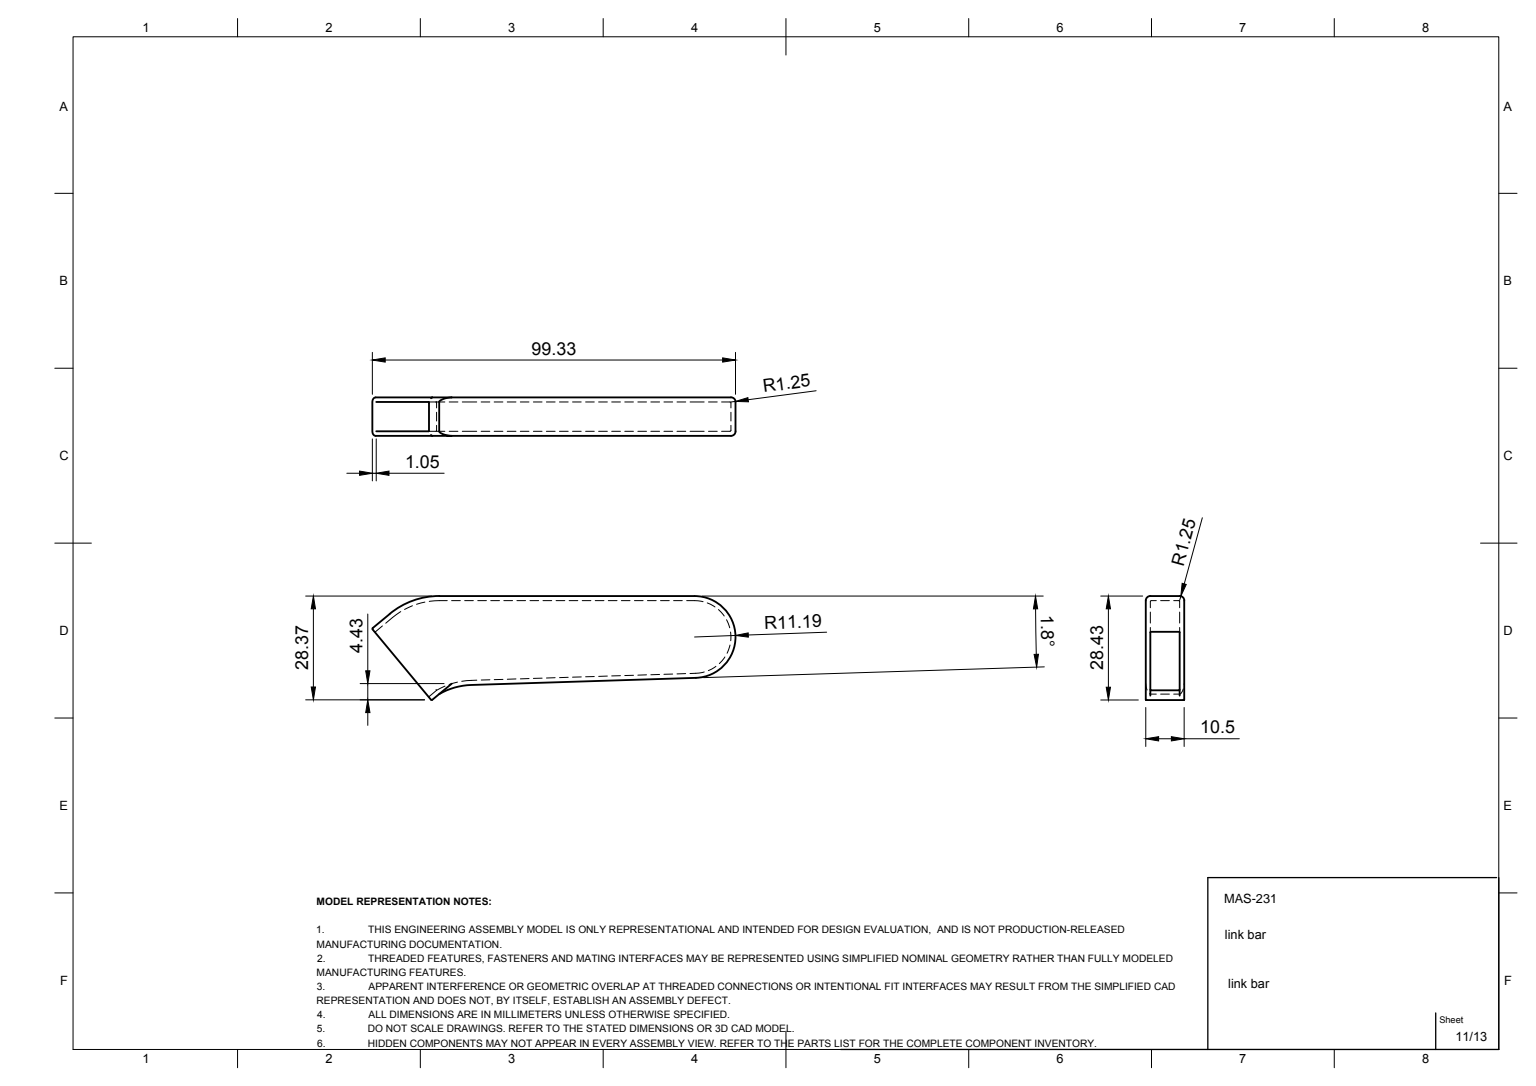
ISO-10303-21;
HEADER;
FILE_DESCRIPTION (('STEP AP214'),
    '1' );
FILE_NAME ( 'Link Bar.step', '2026-10-04T02:08:54', ( '' ), ( '' ), 'STEP AP214', 'Unspecified', '' );
FILE_SCHEMA (( 'AUTOMOTIVE_DESIGN' ));
ENDSEC;
DATA;
#67=ORIENTED_EDGE ( 'NONE', *, *, #18348, .F. ) ;
#85=CARTESIAN_POINT ( 'NONE',  ( 0.1574803149606300023, 0.3648440108500937140, -3.619166627704267558 ) ) ;
#87=CARTESIAN_POINT ( 'NONE',  ( -0.1574803149606299191, 0.7443365962042343131, -3.964450923140766303 ) ) ;
#136=DIRECTION ( 'NONE',  ( -1.000000000000000000, 0.000000000000000000, 0.000000000000000000 ) ) ;
#145=DIRECTION ( 'NONE',  ( 0.000000000000000000, -0.6156614753256641759, -0.7880107536067173513 ) ) ;
#156=DIRECTION ( 'NONE',  ( 0.000000000000000000, 0.6156614753256598460, 0.7880107536067207930 ) ) ;
#159=TOROIDAL_SURFACE ( 'NONE', #46862, 0.3814023619577306956, 0.009842519685039369942 ) ;
#264=EDGE_CURVE ( 'NONE', #24192, #11278, #27216, .T. ) ;
#266=CARTESIAN_POINT ( 'NONE',  ( 0.1673228346456693549, 0.05639690512153990726, -0.1570009270184611616 ) ) ;
#303=EDGE_LOOP ( 'NONE', ( #910, #27362, #9795, #24309 ) ) ;
#308=ORIENTED_EDGE ( 'NONE', *, *, #11008, .T. ) ;
#310=DIRECTION ( 'NONE',  ( 0.000000000000000000, 0.000000000000000000, 1.000000000000000000 ) ) ;
#323=DIRECTION ( 'NONE',  ( -2.602085213965207486E-14, -0.6156614753256566264, -0.7880107536067233465 ) ) ;
#346=CARTESIAN_POINT ( 'NONE',  ( -0.1992661408232795639, -0.3637244504922588773, -1.027838479691305595 ) ) ;
#389=CARTESIAN_POINT ( 'NONE',  ( -0.1673228346456692994, -0.4812165006432425063, -0.8611016091043821596 ) ) ;
#406=DIRECTION ( 'NONE',  ( 0.000000000000000000, -0.2126700594527834443, 0.9771240687918547607 ) ) ;
#428=AXIS2_PLACEMENT_3D ( 'NONE', #42726, #2726, #24548 ) ;
#442=DIRECTION ( 'NONE',  ( 0.000000000000000000, -0.6156614753256597350, -0.7880107536067206819 ) ) ;
#481=ORIENTED_EDGE ( 'NONE', *, *, #44567, .F. ) ;
#483=EDGE_CURVE ( 'NONE', #12524, #45117, #9920, .T. ) ;
#495=FACE_OUTER_BOUND ( 'NONE', #27170, .T. ) ;
#507=CARTESIAN_POINT ( 'NONE',  ( 0.1574803149606300023, -1.308580299410598613, -1.920078980116132872 ) ) ;
#556=DIRECTION ( 'NONE',  ( 0.000000000000000000, 0.9699617890481115889, 0.2432573283306930789 ) ) ;
#568=CARTESIAN_POINT ( 'NONE',  ( -0.2066929133858267931, -0.3022687907404924545, -1.075852903322848331 ) ) ;
#618=DIRECTION ( 'NONE',  ( -0.000000000000000000, 0.7880107536067184615, -0.6156614753256628436 ) ) ;
#643=FACE_OUTER_BOUND ( 'NONE', #21090, .T. ) ;
#670=DIRECTION ( 'NONE',  ( 1.000000000000000000, 0.000000000000000000, -0.000000000000000000 ) ) ;
#700=ORIENTED_EDGE ( 'NONE', *, *, #15382, .F. ) ;
#702=CARTESIAN_POINT ( 'NONE',  ( 0.1925235483212767162, -0.3878655561654137385, -1.008977380820889946 ) ) ;
#751=ORIENTED_EDGE ( 'NONE', *, *, #17520, .F. ) ;
#766=DIRECTION ( 'NONE',  ( -1.000000000000000000, -0.000000000000000000, 0.000000000000000000 ) ) ;
#778=CARTESIAN_POINT ( 'NONE',  ( -0.1476377952755905387, -0.2274162997038010614, -0.9219983537151217323 ) ) ;
#809=CARTESIAN_POINT ( 'NONE',  ( 0.1574803149606300023, 0.06415291647593675262, -0.1630605872086743346 ) ) ;
#816=CARTESIAN_POINT ( 'NONE',  ( -0.1574803149606299191, 0.06415291647593700242, -0.1630605872086743624 ) ) ;
#830=ORIENTED_EDGE ( 'NONE', *, *, #34012, .T. ) ;
#847=EDGE_CURVE ( 'NONE', #7195, #1272, #43787, .T. ) ;
#859=CARTESIAN_POINT ( 'NONE',  ( -0.1673228346456692994, -0.9654866319674424435, -1.480939111413832610 ) ) ;
#860=VERTEX_POINT ( 'NONE', #44704 ) ;
#875=AXIS2_PLACEMENT_3D ( 'NONE', #18309, #25267, #40324 ) ;
#900=AXIS2_PLACEMENT_3D ( 'NONE', #38784, #2573, #27326 ) ;
#910=ORIENTED_EDGE ( 'NONE', *, *, #13077, .T. ) ;
#924=DIRECTION ( 'NONE',  ( 0.000000000000000000, -0.7880107536067184615, 0.6156614753256628436 ) ) ;
#971=DIRECTION ( 'NONE',  ( -1.000000000000000000, 0.000000000000000000, 0.000000000000000000 ) ) ;
#1045=CYLINDRICAL_SURFACE ( 'NONE', #11555, 0.009842519685039274532 ) ;
#1096=CARTESIAN_POINT ( 'NONE',  ( 0.1574803149606300023, -0.4008464425712924273, -0.9238935802775078976 ) ) ;
#1120=ADVANCED_FACE ( 'NONE', ( #44191 ), #22642, .F. ) ;
#1127=DIRECTION ( 'NONE',  ( 0.000000000000000000, -0.2126700594527834443, 0.9771240687918547607 ) ) ;
#1195=AXIS2_PLACEMENT_3D ( 'NONE', #12675, #24382, #42094 ) ;
#1200=EDGE_LOOP ( 'NONE', ( #32073, #12303, #19442, #7739 ) ) ;
#1244=ADVANCED_FACE ( 'NONE', ( #13229 ), #27628, .F. ) ;
#1272=VERTEX_POINT ( 'NONE', #1946 ) ;
#1280=CARTESIAN_POINT ( 'NONE',  ( 0.1574803149606300023, -0.9875035750853327077, -1.463737590216208861 ) ) ;
#1285=CARTESIAN_POINT ( 'NONE',  ( -0.1646842833814627927, -0.4387826116600692661, -0.9691966172188706263 ) ) ;
#1346=DIRECTION ( 'NONE',  ( -0.000000000000000000, 0.7880107536067203489, -0.6156614753256604011 ) ) ;
#1363=CARTESIAN_POINT ( 'NONE',  ( -0.2066929133858267931, 1.174718201258053041, -3.430321324600322797 ) ) ;
#1366=CARTESIAN_POINT ( 'NONE',  ( 0.1476377952755906220, 0.06415291647593697466, -0.1630605872086746122 ) ) ;
#1382=ADVANCED_FACE ( 'NONE', ( #15057 ), #26068, .T. ) ;
#1383=CARTESIAN_POINT ( 'NONE',  ( -0.1574803149606299191, -0.4872761608334555961, -0.8688576204587789009 ) ) ;
#1407=ORIENTED_EDGE ( 'NONE', *, *, #14186, .F. ) ;
#1431=( LENGTH_UNIT ( ) NAMED_UNIT ( * ) SI_UNIT ( $, .METRE. ) ) ;
#1440=ADVANCED_FACE ( 'NONE', ( #26557 ), #44714, .F. ) ;
#1451=AXIS2_PLACEMENT_3D ( 'NONE', #15454, #4626, #8236 ) ;
#1453=ORIENTED_EDGE ( 'NONE', *, *, #37947, .T. ) ;
#1463=( NAMED_UNIT ( * ) PLANE_ANGLE_UNIT ( ) SI_UNIT ( $, .RADIAN. ) ) ;
#1518=CARTESIAN_POINT ( 'NONE',  ( -0.1574803149606299191, 0.3648440108500937140, -3.619166627704267114 ) ) ;
#1554=EDGE_CURVE ( 'NONE', #14871, #42574, #29477, .T. ) ;
#1607=CARTESIAN_POINT ( 'NONE',  ( 0.1574803149606300023, 0.2512968553230416346, -0.3092734567177706229 ) ) ;
#1608=CIRCLE ( 'NONE', #19992, 0.7972440944881888925 ) ;
#1623=DIRECTION ( 'NONE',  ( -1.000000000000000000, -0.000000000000000000, 0.000000000000000000 ) ) ;
#1626=DIRECTION ( 'NONE',  ( 8.439683963172029406E-16, 0.2432573283306645739, -0.9699617890481188054 ) ) ;
#1652=EDGE_LOOP ( 'NONE', ( #44997, #42200, #22401, #33638 ) ) ;
#1681=( CONVERSION_BASED_UNIT ( 'INCH', #5279 ) LENGTH_UNIT ( ) NAMED_UNIT ( #38110 ) ) ;
#1705=DIRECTION ( 'NONE',  ( -0.000000000000000000, 0.7880107536067207930, -0.6156614753256598460 ) ) ;
#1710=ORIENTED_EDGE ( 'NONE', *, *, #13280, .T. ) ;
#1712=FACE_OUTER_BOUND ( 'NONE', #19526, .T. ) ;
#1713=AXIS2_PLACEMENT_3D ( 'NONE', #24114, #35138, #35369 ) ;
#1718=VERTEX_POINT ( 'NONE', #45433 ) ;
#1727=EDGE_CURVE ( 'NONE', #7028, #6659, #38498, .T. ) ;
#1765=ORIENTED_EDGE ( 'NONE', *, *, #13397, .F. ) ;
#1779=ORIENTED_EDGE ( 'NONE', *, *, #33305, .F. ) ;
#1785=CARTESIAN_POINT ( 'NONE',  ( 0.1476377952755906220, -0.4075443641102559078, -0.9311509272141712534 ) ) ;
#1786=TOROIDAL_SURFACE ( 'NONE', #4809, 0.01968503937007873988, 0.009842519685039369942 ) ;
#1853=TOROIDAL_SURFACE ( 'NONE', #17148, 0.7874015748031496509, 0.04921259842519685318 ) ;
#1877=ORIENTED_EDGE ( 'NONE', *, *, #5750, .T. ) ;
#1884=ORIENTED_EDGE ( 'NONE', *, *, #37161, .F. ) ;
#1885=CARTESIAN_POINT ( 'NONE',  ( 0.1574803149606299746, 0.7443365962042343131, -3.523993443072799270 ) ) ;
#1916=AXIS2_PLACEMENT_3D ( 'NONE', #43620, #18692, #26145 ) ;
#1927=DIRECTION ( 'NONE',  ( -1.000000000000000000, -0.000000000000000000, 0.000000000000000000 ) ) ;
#1946=CARTESIAN_POINT ( 'NONE',  ( -0.1574803149606299191, -0.4008464425712929824, -0.9238935802775073425 ) ) ;
#2014=AXIS2_PLACEMENT_3D ( 'NONE', #36944, #44817, #11317 ) ;
#2020=VERTEX_POINT ( 'NONE', #816 ) ;
#2030=ORIENTED_EDGE ( 'NONE', *, *, #1727, .T. ) ;
#2034=CARTESIAN_POINT ( 'NONE',  ( -0.1574803149606299191, -0.4812165006432426173, -0.8611016091043821596 ) ) ;
#2074=ORIENTED_EDGE ( 'NONE', *, *, #27847, .F. ) ;
#2079=FACE_OUTER_BOUND ( 'NONE', #5846, .T. ) ;
#2108=DIRECTION ( 'NONE',  ( 0.000000000000000000, 8.673617379884035472E-16, 1.000000000000000000 ) ) ;
#2198=CARTESIAN_POINT ( 'NONE',  ( 0.1574803149606300023, 0.2573565155132549465, -0.3015174453633734930 ) ) ;
#2203=DIRECTION ( 'NONE',  ( 0.000000000000000000, -0.6156614753256598460, -0.7880107536067207930 ) ) ;
#2238=ORIENTED_EDGE ( 'NONE', *, *, #13233, .T. ) ;
#2256=LINE ( 'NONE', #9473, #8825 ) ;
#2299=ORIENTED_EDGE ( 'NONE', *, *, #37947, .F. ) ;
#2314=DIRECTION ( 'NONE',  ( 1.000000000000000000, 0.000000000000000000, -0.000000000000000000 ) ) ;
#2324=AXIS2_PLACEMENT_3D ( 'NONE', #9453, #24067, #35088 ) ;
#2325=CARTESIAN_POINT ( 'NONE',  ( -0.2066929133858267931, -0.5175744617845221551, -0.9076376772307637175 ) ) ;
#2337=DIRECTION ( 'NONE',  ( 1.000000000000000000, 0.000000000000000000, -0.000000000000000000 ) ) ;
#2341=DIRECTION ( 'NONE',  ( 0.000000000000000000, 0.7880107536067206819, -0.6156614753256597350 ) ) ;
#2360=CARTESIAN_POINT ( 'NONE',  ( 0.1476377952755906220, 0.5419727308409664213, -0.7545416139885205986 ) ) ;
#2371=DIRECTION ( 'NONE',  ( 0.000000000000000000, -0.7880107536067207930, 0.6156614753256597350 ) ) ;
#2375=ORIENTED_EDGE ( 'NONE', *, *, #9641, .T. ) ;
#2418=DIRECTION ( 'NONE',  ( -1.000000000000000000, -0.000000000000000000, -0.000000000000000000 ) ) ;
#2485=ORIENTED_EDGE ( 'NONE', *, *, #8423, .F. ) ;
#2512=CARTESIAN_POINT ( 'NONE',  ( -0.1574803149606299191, -0.2237541348899642346, -1.272196386806234925 ) ) ;
#2521=VERTEX_POINT ( 'NONE', #38786 ) ;
#2548=FACE_OUTER_BOUND ( 'NONE', #14526, .T. ) ;
#2573=DIRECTION ( 'NONE',  ( -1.000000000000000000, -0.000000000000000000, 0.000000000000000000 ) ) ;
#2589=ADVANCED_FACE ( 'NONE', ( #6411 ), #28495, .T. ) ;
#2665=ORIENTED_EDGE ( 'NONE', *, *, #13291, .F. ) ;
#2726=DIRECTION ( 'NONE',  ( 0.000000000000000000, 0.2126700594527845267, -0.9771240687918546497 ) ) ;
#2778=ORIENTED_EDGE ( 'NONE', *, *, #18356, .F. ) ;
#2783=EDGE_CURVE ( 'NONE', #41019, #860, #45985, .T. ) ;
#2788=DIRECTION ( 'NONE',  ( 0.000000000000000000, 0.000000000000000000, 1.000000000000000000 ) ) ;
#2840=DIRECTION ( 'NONE',  ( 1.734723475976806897E-15, -0.6156614753256597350, -0.7880107536067207930 ) ) ;
#2855=VERTEX_POINT ( 'NONE', #30338 ) ;
#2867=VERTEX_POINT ( 'NONE', #44643 ) ;
#2890=ADVANCED_FACE ( 'NONE', ( #15702 ), #1045, .T. ) ;
#2915=CARTESIAN_POINT ( 'NONE',  ( 0.1574803149606300023, 0.7443365962042343131, -3.523993443072799270 ) ) ;
#3014=ORIENTED_EDGE ( 'NONE', *, *, #14197, .T. ) ;
#3025=DIRECTION ( 'NONE',  ( 1.000000000000000000, 0.000000000000000000, -0.000000000000000000 ) ) ;
#3074=DIRECTION ( 'NONE',  ( 0.000000000000000000, 0.7880107536067209040, -0.6156614753256596240 ) ) ;
#3086=EDGE_CURVE ( 'NONE', #23115, #28092, #1608, .T. ) ;
#3090=DIRECTION ( 'NONE',  ( 0.000000000000000000, 0.000000000000000000, 1.000000000000000000 ) ) ;
#3113=ORIENTED_EDGE ( 'NONE', *, *, #40975, .F. ) ;
#3125=CARTESIAN_POINT ( 'NONE',  ( -0.2066929133858267931, 0.1005108776172154716, -0.1165245190822937899 ) ) ;
#3141=CIRCLE ( 'NONE', #35331, 0.01968503937007870172 ) ;
#3153=FACE_OUTER_BOUND ( 'NONE', #4062, .T. ) ;
#3170=CARTESIAN_POINT ( 'NONE',  ( 0.1968503937007874682, -0.5192708129487058066, -0.8938220056861535534 ) ) ;
#3201=ORIENTED_EDGE ( 'NONE', *, *, #36095, .T. ) ;
#3203=EDGE_LOOP ( 'NONE', ( #24466, #16321, #10489, #24480 ) ) ;
#3232=ORIENTED_EDGE ( 'NONE', *, *, #31414, .F. ) ;
#3254=EDGE_CURVE ( 'NONE', #6831, #11278, #11439, .T. ) ;
#3262=ORIENTED_EDGE ( 'NONE', *, *, #4046, .T. ) ;
#3385=PLANE ( 'NONE',  #24870 ) ;
#3432=DIRECTION ( 'NONE',  ( 0.000000000000000000, -0.6156614753256597350, -0.7880107536067207930 ) ) ;
#3564=CARTESIAN_POINT ( 'NONE',  ( 0.2026160082443593247, -0.5228204797047603103, -0.8983653719476394350 ) ) ;
#3570=ORIENTED_EDGE ( 'NONE', *, *, #1554, .T. ) ;
#3584=DIRECTION ( 'NONE',  ( 0.000000000000000000, -0.6156614753256597350, -0.7880107536067207930 ) ) ;
#3598=CARTESIAN_POINT ( 'NONE',  ( -0.1476377952755905387, -0.2237541348899636795, -1.272196386806235813 ) ) ;
#3621=ORIENTED_EDGE ( 'NONE', *, *, #35353, .T. ) ;
#3627=ADVANCED_FACE ( 'NONE', ( #9726 ), #9493, .F. ) ;
#3635=CARTESIAN_POINT ( 'NONE',  ( 0.1574803149606300023, 1.126631386849005878, -3.440787370833236380 ) ) ;
#3681=CARTESIAN_POINT ( 'NONE',  ( 0.1476377952755906220, 0.7443365962042343131, -3.523993443072799270 ) ) ;
#3703=CARTESIAN_POINT ( 'NONE',  ( -0.2066929133858267931, 1.126631386849004990, -3.440787370833234604 ) ) ;
#3729=ORIENTED_EDGE ( 'NONE', *, *, #1554, .F. ) ;
#3733=ADVANCED_FACE ( 'NONE', ( #495 ), #30907, .T. ) ;
#3741=ADVANCED_FACE ( 'NONE', ( #38301 ), #12924, .F. ) ;
#3747=EDGE_LOOP ( 'NONE', ( #10577, #3201, #42550, #19624 ) ) ;
#3763=CARTESIAN_POINT ( 'NONE',  ( 0.1574803149606300023, 0.3743908788525355247, -3.616772362661642148 ) ) ;
#3767=ORIENTED_EDGE ( 'NONE', *, *, #37986, .T. ) ;
#3771=CARTESIAN_POINT ( 'NONE',  ( -0.2066929133858267931, -0.5175744617845221551, -0.9076376772307634955 ) ) ;
#3845=EDGE_LOOP ( 'NONE', ( #17687, #36233, #28151, #41572 ) ) ;
#3901=EDGE_LOOP ( 'NONE', ( #21553, #3621, #40491, #10280 ) ) ;
#3908=ORIENTED_EDGE ( 'NONE', *, *, #23614, .T. ) ;
#3972=EDGE_LOOP ( 'NONE', ( #24578, #14128, #46856, #40143 ) ) ;
#4046=EDGE_CURVE ( 'NONE', #28221, #6310, #37272, .T. ) ;
#4062=EDGE_LOOP ( 'NONE', ( #22601, #3570, #16300, #5663 ) ) ;
#4071=DIRECTION ( 'NONE',  ( 1.000000000000000000, 0.000000000000000000, 0.000000000000000000 ) ) ;
#4073=CARTESIAN_POINT ( 'NONE',  ( -0.1476377952755905387, -0.4889725119976395251, -0.8550419489141688478 ) ) ;
#4126=ORIENTED_EDGE ( 'NONE', *, *, #29729, .F. ) ;
#4140=FACE_OUTER_BOUND ( 'NONE', #39147, .T. ) ;
#4154=CIRCLE ( 'NONE', #8875, 0.04921259842519691563 ) ;
#4163=LINE ( 'NONE', #19012, #46583 ) ;
#4218=TOROIDAL_SURFACE ( 'NONE', #9594, 0.01968503937007873988, 0.009842519685039369942 ) ;
#4236=CARTESIAN_POINT ( 'NONE',  ( 0.2066929133858267653, -0.5221178280460081478, -0.9040880104747088808 ) ) ;
#4265=CARTESIAN_POINT ( 'NONE',  ( -0.1574803149606299191, 0.3171096708378827178, -3.631137952917390166 ) ) ;
#4278=LINE ( 'NONE', #30688, #6833 ) ;
#4385=DIRECTION ( 'NONE',  ( -0.000000000000000000, -0.7880107536067200158, 0.6156614753256608452 ) ) ;
#4396=CARTESIAN_POINT ( 'NONE',  ( -0.1613934693438489332, -0.4404989748867991217, -0.9678556472999616522 ) ) ;
#4444=FACE_OUTER_BOUND ( 'NONE', #303, .T. ) ;
#4499=DIRECTION ( 'NONE',  ( 0.000000000000000000, -0.7880107536067207930, 0.6156614753256598460 ) ) ;
#4539=ORIENTED_EDGE ( 'NONE', *, *, #21973, .T. ) ;
#4546=ORIENTED_EDGE ( 'NONE', *, *, #46961, .F. ) ;
#4555=CIRCLE ( 'NONE', #9964, 0.04921259842519686706 ) ;
#4598=ORIENTED_EDGE ( 'NONE', *, *, #7307, .F. ) ;
#4624=EDGE_LOOP ( 'NONE', ( #6787, #17164, #42331, #39743 ) ) ;
#4626=DIRECTION ( 'NONE',  ( 2.263915770909195608E-15, -0.6156614753256604011, -0.7880107536067204599 ) ) ;
#4629=ADVANCED_FACE ( 'NONE', ( #45517 ), #5760, .F. ) ;
#4651=ADVANCED_FACE ( 'NONE', ( #9121 ), #1853, .T. ) ;
#4655=CIRCLE ( 'NONE', #23032, 0.009842519685039363003 ) ;
#4709=ORIENTED_EDGE ( 'NONE', *, *, #13004, .F. ) ;
#4742=CIRCLE ( 'NONE', #19299, 0.3814023619577306956 ) ;
#4809=AXIS2_PLACEMENT_3D ( 'NONE', #31422, #23988, #16554 ) ;
#4855=EDGE_CURVE ( 'NONE', #2020, #6624, #40085, .T. ) ;
#4879=DIRECTION ( 'NONE',  ( 1.000000000000000000, 0.000000000000000000, -0.000000000000000000 ) ) ;
#4885=CARTESIAN_POINT ( 'NONE',  ( -0.2066929133858267653, -0.3147020779469855145, -1.066138954738185651 ) ) ;
#4896=DIRECTION ( 'NONE',  ( -1.000000000000000000, -0.000000000000000000, 0.000000000000000000 ) ) ;
#4938=CYLINDRICAL_SURFACE ( 'NONE', #26938, 0.009842519685039382085 ) ;
#4947=DIRECTION ( 'NONE',  ( 0.000000000000000000, -0.9699617890481186944, -0.2432573283306648515 ) ) ;
#4967=EDGE_CURVE ( 'NONE', #46334, #2521, #21777, .T. ) ;
#4983=AXIS2_PLACEMENT_3D ( 'NONE', #45204, #30190, #41841 ) ;
#4992=CARTESIAN_POINT ( 'NONE',  ( -0.2066929133858267931, 0.09275486626281861935, -0.1104648588920805335 ) ) ;
#5023=FACE_OUTER_BOUND ( 'NONE', #22860, .T. ) ;
#5042=( NAMED_UNIT ( * ) PLANE_ANGLE_UNIT ( ) SI_UNIT ( $, .RADIAN. ) ) ;
#5046=CARTESIAN_POINT ( 'NONE',  ( -0.1476377952755905387, -0.9875035750853327077, -1.463737590216208861 ) ) ;
#5132=VERTEX_POINT ( 'NONE', #37824 ) ;
#5140=ORIENTED_EDGE ( 'NONE', *, *, #18243, .T. ) ;
#5143=ADVANCED_FACE ( 'NONE', ( #16495 ), #27981, .F. ) ;
#5169=CARTESIAN_POINT ( 'NONE',  ( 0.1574803149606307795, -0.4026036378687909423, -0.9257984838013391116 ) ) ;
#5173=LINE ( 'NONE', #15756, #16894 ) ;
#5180=VERTEX_POINT ( 'NONE', #38054 ) ;
#5196=DIRECTION ( 'NONE',  ( 0.000000000000000000, -0.6156614753256597350, -0.7880107536067206819 ) ) ;
#5219=CARTESIAN_POINT ( 'NONE',  ( 0.1476377952755906220, -0.2274162997038010614, -0.9219983537151217323 ) ) ;
#5246=VERTEX_POINT ( 'NONE', #31593 ) ;
#5256=EDGE_CURVE ( 'NONE', #47128, #1718, #46309, .T. ) ;
#5279=LENGTH_MEASURE_WITH_UNIT ( LENGTH_MEASURE( 0.02539999999999999897 ), #1431 ) ;
#5286=LINE ( 'NONE', #37402, #15486 ) ;
#5338=FACE_OUTER_BOUND ( 'NONE', #16104, .T. ) ;
#5376=CIRCLE ( 'NONE', #31510, 0.009842519685039387289 ) ;
#5387=EDGE_CURVE ( 'NONE', #44611, #5246, #22575, .T. ) ;
#5420=ORIENTED_EDGE ( 'NONE', *, *, #14186, .T. ) ;
#5435=VERTEX_POINT ( 'NONE', #18170 ) ;
#5475=CARTESIAN_POINT ( 'NONE',  ( 0.1574803149606300023, 1.117014023967196401, -3.442880580079819008 ) ) ;
#5574=ADVANCED_FACE ( 'NONE', ( #1712 ), #9399, .T. ) ;
#5663=ORIENTED_EDGE ( 'NONE', *, *, #23020, .T. ) ;
#5690=ADVANCED_FACE ( 'NONE', ( #32644 ), #14414, .F. ) ;
#5717=AXIS2_PLACEMENT_3D ( 'NONE', #14443, #6526, #25482 ) ;
#5747=CARTESIAN_POINT ( 'NONE',  ( 0.2066929133858268486, 0.06245656531175283743, -0.1492449156640649477 ) ) ;
#5750=EDGE_CURVE ( 'NONE', #5132, #42574, #30242, .T. ) ;
#5753=ORIENTED_EDGE ( 'NONE', *, *, #23116, .T. ) ;
#5760=CYLINDRICAL_SURFACE ( 'NONE', #27135, 0.009842519685039387289 ) ;
#5804=LINE ( 'NONE', #2198, #15871 ) ;
#5830=LINE ( 'NONE', #20437, #14580 ) ;
#5846=EDGE_LOOP ( 'NONE', ( #25452, #3729, #12691, #15112 ) ) ;
#5924=CARTESIAN_POINT ( 'NONE',  ( -0.1968503937007874127, -0.5192708129487058066, -0.8938220056861535534 ) ) ;
#5950=SHAPE_REPRESENTATION ( 'Link Bar', ( #20860 ), #6323 ) ;
#6004=DIRECTION ( 'NONE',  ( -1.000000000000000000, -0.000000000000000000, 0.000000000000000000 ) ) ;
#6021=AXIS2_PLACEMENT_3D ( 'NONE', #45675, #23431, #22951 ) ;
#6044=DIRECTION ( 'NONE',  ( 1.000000000000000000, -0.000000000000000000, -0.000000000000000000 ) ) ;
#6047=EDGE_LOOP ( 'NONE', ( #7657, #28457, #38794, #28639, #23318 ) ) ;
#6117=DIRECTION ( 'NONE',  ( 0.000000000000000000, -0.9771240687918510970, -0.2126700594528006527 ) ) ;
#6124=VERTEX_POINT ( 'NONE', #43273 ) ;
#6137=CYLINDRICAL_SURFACE ( 'NONE', #33351, 0.4404574800679669777 ) ;
#6213=VECTOR ( 'NONE', #36585, 39.37007874015748143 ) ;
#6236=LINE ( 'NONE', #35273, #14392 ) ;
#6310=VERTEX_POINT ( 'NONE', #44438 ) ;
#6323=( GEOMETRIC_REPRESENTATION_CONTEXT ( 3 ) GLOBAL_UNCERTAINTY_ASSIGNED_CONTEXT ( ( #40306 ) ) GLOBAL_UNIT_ASSIGNED_CONTEXT ( ( #1681, #5042, #12502 ) ) REPRESENTATION_CONTEXT ( 'NONE', 'WORKASPACE' ) ) ;
#6330=EDGE_CURVE ( 'NONE', #23068, #47303, #2256, .T. ) ;
#6409=DIRECTION ( 'NONE',  ( 0.000000000000000000, 0.000000000000000000, 1.000000000000000000 ) ) ;
#6411=FACE_OUTER_BOUND ( 'NONE', #14762, .T. ) ;
#6526=DIRECTION ( 'NONE',  ( -9.133235551360036525E-15, 0.2126700594527874688, -0.9771240687918542056 ) ) ;
#6624=VERTEX_POINT ( 'NONE', #16949 ) ;
#6650=DIRECTION ( 'NONE',  ( 0.000000000000000000, 0.000000000000000000, 1.000000000000000000 ) ) ;
#6652=ORIENTED_EDGE ( 'NONE', *, *, #30354, .F. ) ;
#6659=VERTEX_POINT ( 'NONE', #42085 ) ;
#6661=ORIENTED_EDGE ( 'NONE', *, *, #10572, .T. ) ;
#6706=CARTESIAN_POINT ( 'NONE',  ( 0.1574803149606299746, 0.2876548164643190630, -0.2627373885913885099 ) ) ;
#6722=DIRECTION ( 'NONE',  ( -1.000000000000000000, -0.000000000000000000, 0.000000000000000000 ) ) ;
#6725=ORIENTED_EDGE ( 'NONE', *, *, #14530, .F. ) ;
#6729=CARTESIAN_POINT ( 'NONE',  ( -0.1574803149606299191, 0.07021257666614952320, -0.1553045758542780375 ) ) ;
#6787=ORIENTED_EDGE ( 'NONE', *, *, #18184, .T. ) ;
#6831=VERTEX_POINT ( 'NONE', #17409 ) ;
#6833=VECTOR ( 'NONE', #41165, 39.37007874015748854 ) ;
#6990=DIRECTION ( 'NONE',  ( 0.000000000000000000, -0.2126700594527834443, 0.9771240687918547607 ) ) ;
#7023=CARTESIAN_POINT ( 'NONE',  ( -0.1476377952755905387, -0.4812165006432426728, -0.8611016091043821596 ) ) ;
#7028=VERTEX_POINT ( 'NONE', #44447 ) ;
#7107=LINE ( 'NONE', #21964, #6213 ) ;
#7160=EDGE_CURVE ( 'NONE', #28305, #6831, #4154, .T. ) ;
#7195=VERTEX_POINT ( 'NONE', #2034 ) ;
#7307=EDGE_CURVE ( 'NONE', #6310, #19153, #31093, .T. ) ;
#7315=EDGE_CURVE ( 'NONE', #47128, #14871, #15017, .T. ) ;
#7372=CARTESIAN_POINT ( 'NONE',  ( 0.1574803149606300023, 0.08669520607260541856, -0.1182208702464773997 ) ) ;
#7498=ORIENTED_EDGE ( 'NONE', *, *, #34709, .T. ) ;
#7500=AXIS2_PLACEMENT_3D ( 'NONE', #31272, #31973, #42485 ) ;
#7550=VERTEX_POINT ( 'NONE', #36986 ) ;
#7570=TOROIDAL_SURFACE ( 'NONE', #6021, 0.7775590551181102983, 0.009842519685039369942 ) ;
#7643=DIRECTION ( 'NONE',  ( -0.000000000000000000, 0.6156614753256597350, 0.7880107536067206819 ) ) ;
#7657=ORIENTED_EDGE ( 'NONE', *, *, #7160, .T. ) ;
#7712=CARTESIAN_POINT ( 'NONE',  ( 0.1476377952755906220, 1.571700394971587755, -2.465016072061059660 ) ) ;
#7739=ORIENTED_EDGE ( 'NONE', *, *, #38350, .T. ) ;
#7743=DIRECTION ( 'NONE',  ( 1.000000000000000000, 0.000000000000000000, 0.000000000000000000 ) ) ;
#7775=CARTESIAN_POINT ( 'NONE',  ( -0.1720110121816429416, -0.4314947915448568705, -0.9748904863234528761 ) ) ;
#7796=TOROIDAL_SURFACE ( 'NONE', #18505, 0.7874015748031495399, 0.04921259842519685318 ) ;
#7809=PRODUCT_DEFINITION ( 'UNKNOWN', '', #30151, #29373 ) ;
#7833=AXIS2_PLACEMENT_3D ( 'NONE', #45772, #34091, #34320 ) ;
#7852=DIRECTION ( 'NONE',  ( 0.000000000000000000, -0.7880107536067200158, 0.6156614753256607342 ) ) ;
#7917=CARTESIAN_POINT ( 'NONE',  ( 0.1700368126712054895, -0.4340694319687135039, -0.9728789567668699734 ) ) ;
#7930=B_SPLINE_CURVE_WITH_KNOTS ( 'NONE', 3,
 ( #30639, #26566, #30185, #41123, #40339, #44639 ),
 .UNSPECIFIED., .F., .F.,
 ( 4, 2, 4 ),
 ( 0.000000000000000000, 0.0001956124598869668702, 0.0003912249197739337404 ),
 .UNSPECIFIED. ) ;
#8003=CARTESIAN_POINT ( 'NONE',  ( 0.1476377952755906220, 0.4814845645395590679, -0.4766254685646189593 ) ) ;
#8010=CARTESIAN_POINT ( 'NONE',  ( -0.1574803149606299191, -0.4410959923581754816, -0.9673892061308019263 ) ) ;
#8018=LINE ( 'NONE', #43489, #13951 ) ;
#8035=EDGE_LOOP ( 'NONE', ( #1710, #3014, #36563, #34820, #10818, #44347 ) ) ;
#8087=CARTESIAN_POINT ( 'NONE',  ( 0.1968503937007874682, -0.5192708129487058066, -0.8938220056861535534 ) ) ;
#8138=DIRECTION ( 'NONE',  ( -1.000000000000000000, -0.000000000000000000, 0.000000000000000000 ) ) ;
#8236=DIRECTION ( 'NONE',  ( 0.000000000000000000, 0.7880107536067200158, -0.6156614753256607342 ) ) ;
#8267=ORIENTED_EDGE ( 'NONE', *, *, #30354, .T. ) ;
#8303=ADVANCED_FACE ( 'NONE', ( #40490 ), #3385, .T. ) ;
#8316=VECTOR ( 'NONE', #13814, 39.37007874015748143 ) ;
#8318=DIRECTION ( 'NONE',  ( 0.000000000000000000, -0.7880107536067207930, 0.6156614753256598460 ) ) ;
#8320=DIRECTION ( 'NONE',  ( -1.000000000000000000, -0.000000000000000000, 0.000000000000000000 ) ) ;
#8350=CYLINDRICAL_SURFACE ( 'NONE', #42905, 0.009842519685039286675 ) ;
#8378=VECTOR ( 'NONE', #27140, 39.37007874015748854 ) ;
#8383=CARTESIAN_POINT ( 'NONE',  ( -0.1476377952755905387, 0.06851622550196635741, -0.1414889043096673460 ) ) ;
#8389=AXIS2_PLACEMENT_3D ( 'NONE', #10279, #39485, #46918 ) ;
#8405=VECTOR ( 'NONE', #406, 39.37007874015748854 ) ;
#8423=EDGE_CURVE ( 'NONE', #29301, #5246, #44713, .T. ) ;
#8451=CARTESIAN_POINT ( 'NONE',  ( -0.2066929133858267931, -0.2237541348899642346, -1.272196386806234925 ) ) ;
#8476=DIRECTION ( 'NONE',  ( 0.000000000000000000, -0.7880107536067184615, 0.6156614753256628436 ) ) ;
#8482=CARTESIAN_POINT ( 'NONE',  ( -0.1699495073158193426, -0.4341647314679547565, -0.9728045006378999160 ) ) ;
#8494=AXIS2_PLACEMENT_3D ( 'NONE', #24924, #21803, #3584 ) ;
#8495=VERTEX_POINT ( 'NONE', #1785 ) ;
#8533=DIRECTION ( 'NONE',  ( -1.000000000000000000, -0.000000000000000000, 0.000000000000000000 ) ) ;
#8560=LINE ( 'NONE', #38039, #32846 ) ;
#8594=CARTESIAN_POINT ( 'NONE',  ( -0.1476377952755905387, 0.07627223685636332073, -0.1475485644998805745 ) ) ;
#8597=VERTEX_POINT ( 'NONE', #11777 ) ;
#8682=ORIENTED_EDGE ( 'NONE', *, *, #23020, .F. ) ;
#8699=EDGE_CURVE ( 'NONE', #860, #25910, #35000, .T. ) ;
#8736=ORIENTED_EDGE ( 'NONE', *, *, #22775, .T. ) ;
#8809=VECTOR ( 'NONE', #924, 39.37007874015748143 ) ;
#8824=FACE_OUTER_BOUND ( 'NONE', #10383, .T. ) ;
#8825=VECTOR ( 'NONE', #27932, 39.37007874015748854 ) ;
#8875=AXIS2_PLACEMENT_3D ( 'NONE', #35351, #27478, #42029 ) ;
#8915=ORIENTED_EDGE ( 'NONE', *, *, #34012, .F. ) ;
#8943=CIRCLE ( 'NONE', #15084, 0.009842519685039376881 ) ;
#8964=VERTEX_POINT ( 'NONE', #28764 ) ;
#8992=VERTEX_POINT ( 'NONE', #10294 ) ;
#8998=EDGE_CURVE ( 'NONE', #28190, #45599, #35622, .T. ) ;
#9036=EDGE_CURVE ( 'NONE', #45117, #41157, #19530, .T. ) ;
#9074=DIRECTION ( 'NONE',  ( -1.000000000000000000, -0.000000000000000000, 0.000000000000000000 ) ) ;
#9121=FACE_OUTER_BOUND ( 'NONE', #21012, .T. ) ;
#9167=ORIENTED_EDGE ( 'NONE', *, *, #19719, .T. ) ;
#9169=CARTESIAN_POINT ( 'NONE',  ( -0.1476377952755905387, 0.06415291647593691915, -0.1630605872086743346 ) ) ;
#9177=ADVANCED_FACE ( 'NONE', ( #22473 ), #4218, .T. ) ;
#9258=ADVANCED_FACE ( 'NONE', ( #643 ), #15789, .T. ) ;
#9316=AXIS2_PLACEMENT_3D ( 'NONE', #15688, #19252, #25590 ) ;
#9358=AXIS2_PLACEMENT_3D ( 'NONE', #28001, #13588, #10249 ) ;
#9359=CIRCLE ( 'NONE', #16274, 0.01968503937007874335 ) ;
#9370=EDGE_CURVE ( 'NONE', #5180, #25679, #5804, .T. ) ;
#9375=ORIENTED_EDGE ( 'NONE', *, *, #32024, .T. ) ;
#9399=CYLINDRICAL_SURFACE ( 'NONE', #23345, 0.7874015748031495399 ) ;
#9453=CARTESIAN_POINT ( 'NONE',  ( 0.1574803149606300023, -0.2237541348899636795, -1.272196386806235813 ) ) ;
#9473=CARTESIAN_POINT ( 'NONE',  ( -0.1673228346456692994, 0.06245656531175331622, -0.1492449156640640040 ) ) ;
#9478=VERTEX_POINT ( 'NONE', #34572 ) ;
#9493=CYLINDRICAL_SURFACE ( 'NONE', #1713, 0.3912448816427701037 ) ;
#9520=ORIENTED_EDGE ( 'NONE', *, *, #21130, .T. ) ;
#9557=DIRECTION ( 'NONE',  ( 0.000000000000000000, 0.000000000000000000, 1.000000000000000000 ) ) ;
#9561=FACE_OUTER_BOUND ( 'NONE', #20700, .T. ) ;
#9594=AXIS2_PLACEMENT_3D ( 'NONE', #1366, #16020, #41126 ) ;
#9603=FACE_OUTER_BOUND ( 'NONE', #3747, .T. ) ;
#9641=EDGE_CURVE ( 'NONE', #1718, #5180, #8943, .T. ) ;
#9649=VECTOR ( 'NONE', #1346, 39.37007874015748143 ) ;
#9650=CARTESIAN_POINT ( 'NONE',  ( 0.1476377952755906220, -0.5010918323780657602, -0.8705539716229625524 ) ) ;
#9726=FACE_OUTER_BOUND ( 'NONE', #29954, .T. ) ;
#9733=CARTESIAN_POINT ( 'NONE',  ( -0.1476377952755905387, -0.2237541348899639571, -1.272196386806235813 ) ) ;
#9790=CARTESIAN_POINT ( 'NONE',  ( -0.1574803149606299191, -0.9875035750853327077, -1.463737590216208861 ) ) ;
#9795=ORIENTED_EDGE ( 'NONE', *, *, #18705, .F. ) ;
#9799=DIRECTION ( 'NONE',  ( 0.000000000000000000, 0.000000000000000000, 1.000000000000000000 ) ) ;
#9810=ORIENTED_EDGE ( 'NONE', *, *, #39428, .T. ) ;
#9866=CARTESIAN_POINT ( 'NONE',  ( -0.1476377952755905387, 0.3648440108500937140, -3.619166627704267558 ) ) ;
#9920=LINE ( 'NONE', #21643, #21001 ) ;
#9964=AXIS2_PLACEMENT_3D ( 'NONE', #44477, #33280, #4947 ) ;
#9999=ORIENTED_EDGE ( 'NONE', *, *, #45991, .F. ) ;
#10065=COLOUR_RGB ( '', 0.31764706, 0.68627451, 0.89019608) ;
#10093=CIRCLE ( 'NONE', #36871, 0.009842519685039382085 ) ;
#10110=EDGE_LOOP ( 'NONE', ( #18965, #34973, #46917, #11242, #12130, #14378, #16039, #23716 ) ) ;
#10132=DIRECTION ( 'NONE',  ( 0.000000000000000000, 0.000000000000000000, -1.000000000000000000 ) ) ;
#10139=CIRCLE ( 'NONE', #43786, 0.3814023619577306956 ) ;
#10147=DIRECTION ( 'NONE',  ( 0.000000000000000000, -0.7880107536067207930, 0.6156614753256598460 ) ) ;
#10177=EDGE_LOOP ( 'NONE', ( #40262, #3767, #11982, #12660 ) ) ;
#10192=CARTESIAN_POINT ( 'NONE',  ( -0.2066929133858267931, 0.08669520607260541856, -0.1182208702464773997 ) ) ;
#10249=DIRECTION ( 'NONE',  ( 0.000000000000000000, 0.000000000000000000, 1.000000000000000000 ) ) ;
#10256=ORIENTED_EDGE ( 'NONE', *, *, #31779, .F. ) ;
#10275=ORIENTED_EDGE ( 'NONE', *, *, #33628, .F. ) ;
#10279=CARTESIAN_POINT ( 'NONE',  ( -0.1476377952755905387, -0.2274162997038010614, -0.9219983537151217323 ) ) ;
#10280=ORIENTED_EDGE ( 'NONE', *, *, #22414, .T. ) ;
#10294=CARTESIAN_POINT ( 'NONE',  ( 0.2066929133858268486, -0.3022687907404924545, -1.075852903322848331 ) ) ;
#10295=DIRECTION ( 'NONE',  ( 0.000000000000000000, -0.6156614753256598460, -0.7880107536067207930 ) ) ;
#10357=CARTESIAN_POINT ( 'NONE',  ( -0.1574803149606299191, 0.7443365962042343131, -3.523993443072799270 ) ) ;
#10369=CARTESIAN_POINT ( 'NONE',  ( 0.1476377952755906220, -0.4872761608334559846, -0.8688576204587790119 ) ) ;
#10383=EDGE_LOOP ( 'NONE', ( #3908, #1884, #46345, #35752 ) ) ;
#10421=AXIS2_PLACEMENT_3D ( 'NONE', #778, #15437, #2788 ) ;
#10465=ORIENTED_EDGE ( 'NONE', *, *, #39731, .F. ) ;
#10489=ORIENTED_EDGE ( 'NONE', *, *, #9370, .T. ) ;
#10554=VERTEX_POINT ( 'NONE', #37740 ) ;
#10565=ORIENTED_EDGE ( 'NONE', *, *, #37045, .T. ) ;
#10572=EDGE_CURVE ( 'NONE', #46402, #43921, #23530, .T. ) ;
#10577=ORIENTED_EDGE ( 'NONE', *, *, #42871, .T. ) ;
#10611=PLANE ( 'NONE',  #19599 ) ;
#10676=CARTESIAN_POINT ( 'NONE',  ( -0.1476377952755905387, 0.3743908788525359133, -3.616772362661642592 ) ) ;
#10699=ORIENTED_EDGE ( 'NONE', *, *, #27847, .T. ) ;
#10707=ORIENTED_EDGE ( 'NONE', *, *, #15433, .F. ) ;
#10811=AXIS2_PLACEMENT_3D ( 'NONE', #13382, #2337, #23931 ) ;
#10818=ORIENTED_EDGE ( 'NONE', *, *, #19148, .T. ) ;
#10835=DIRECTION ( 'NONE',  ( 1.000000000000000000, 0.000000000000000000, 0.000000000000000000 ) ) ;
#10895=ORIENTED_EDGE ( 'NONE', *, *, #9370, .F. ) ;
#10900=AXIS2_PLACEMENT_3D ( 'NONE', #43405, #24507, #10132 ) ;
#10968=CARTESIAN_POINT ( 'NONE',  ( 0.1673228346456693549, -0.4889725119976396361, -0.8550419489141689589 ) ) ;
#11001=CARTESIAN_POINT ( 'NONE',  ( -0.1574803149606299191, 0.5323553679591568333, -0.7566348232351034486 ) ) ;
#11008=EDGE_CURVE ( 'NONE', #28092, #30092, #26722, .T. ) ;
#11023=ORIENTED_EDGE ( 'NONE', *, *, #34924, .F. ) ;
#11064=CARTESIAN_POINT ( 'NONE',  ( 0.2066929133858268486, -0.3146900525635061840, -1.066148349997451339 ) ) ;
#11075=FACE_OUTER_BOUND ( 'NONE', #45725, .T. ) ;
#11159=ORIENTED_EDGE ( 'NONE', *, *, #12423, .F. ) ;
#11225=ORIENTED_EDGE ( 'NONE', *, *, #35353, .F. ) ;
#11242=ORIENTED_EDGE ( 'NONE', *, *, #33628, .T. ) ;
#11264=LINE ( 'NONE', #44761, #28486 ) ;
#11278=VERTEX_POINT ( 'NONE', #35333 ) ;
#11294=CARTESIAN_POINT ( 'NONE',  ( 0.1776748150188054431, -0.4231595423373736287, -0.9814026967226106013 ) ) ;
#11303=ADVANCED_FACE ( 'NONE', ( #38442 ), #39365, .F. ) ;
#11317=DIRECTION ( 'NONE',  ( 0.000000000000000000, 0.000000000000000000, 1.000000000000000000 ) ) ;
#11318=DIRECTION ( 'NONE',  ( 0.000000000000000000, 0.000000000000000000, -1.000000000000000000 ) ) ;
#11334=ORIENTED_EDGE ( 'NONE', *, *, #21603, .F. ) ;
#11386=CARTESIAN_POINT ( 'NONE',  ( 0.1968503937007874682, -1.308580299410598613, -1.920078980116132872 ) ) ;
#11390=CARTESIAN_POINT ( 'NONE',  ( -0.2019004115846159131, -0.3515432751093511277, -1.037355456931929210 ) ) ;
#11418=CIRCLE ( 'NONE', #15256, 0.009842519685039369942 ) ;
#11420=DIRECTION ( 'NONE',  ( -1.000000000000000000, -0.000000000000000000, 0.000000000000000000 ) ) ;
#11427=DIRECTION ( 'NONE',  ( 0.000000000000000000, 0.000000000000000000, 1.000000000000000000 ) ) ;
#11439=LINE ( 'NONE', #29228, #27771 ) ;
#11448=CARTESIAN_POINT ( 'NONE',  ( -0.1574803149606299191, 0.7443365962042343131, -3.523993443072799270 ) ) ;
#11517=DIRECTION ( 'NONE',  ( 0.000000000000000000, 0.000000000000000000, -1.000000000000000000 ) ) ;
#11527=CARTESIAN_POINT ( 'NONE',  ( 0.1885137525767837108, -0.3997902715136080753, -0.9996607721191614893 ) ) ;
#11555=AXIS2_PLACEMENT_3D ( 'NONE', #11386, #37013, #15461 ) ;
#11556=DIRECTION ( 'NONE',  ( 0.000000000000000000, 0.000000000000000000, 1.000000000000000000 ) ) ;
#11572=FACE_OUTER_BOUND ( 'NONE', #1200, .T. ) ;
#11606=PRODUCT_CONTEXT ( 'NONE', #15971, 'mechanical' ) ;
#11608=TOROIDAL_SURFACE ( 'NONE', #25369, 0.3912448816427699927, 0.04921259842519685318 ) ;
#11632=FACE_OUTER_BOUND ( 'NONE', #28011, .T. ) ;
#11664=AXIS2_PLACEMENT_3D ( 'NONE', #9169, #23557, #2203 ) ;
#11688=VECTOR ( 'NONE', #15164, 39.37007874015748854 ) ;
#11700=EDGE_CURVE ( 'NONE', #8495, #5435, #6236, .T. ) ;
#11704=DIRECTION ( 'NONE',  ( 0.000000000000000000, -0.6156614753256598460, -0.7880107536067206819 ) ) ;
#11758=CARTESIAN_POINT ( 'NONE',  ( 0.1614206436753637397, -0.4404907083123212330, -0.9678621058557815848 ) ) ;
#11763=CARTESIAN_POINT ( 'NONE',  ( 0.1574803149606300023, 0.07627223685636330686, -0.1475485644998806023 ) ) ;
#11777=CARTESIAN_POINT ( 'NONE',  ( 0.1476377952755906220, 0.3648440108500937140, -3.619166627704267558 ) ) ;
#11853=DIRECTION ( 'NONE',  ( -1.000000000000000000, -0.000000000000000000, 0.000000000000000000 ) ) ;
#11873=LINE ( 'NONE', #34869, #32355 ) ;
#11895=CIRCLE ( 'NONE', #27197, 0.3912448816427701037 ) ;
#11896=AXIS2_PLACEMENT_3D ( 'NONE', #42095, #12191, #31125 ) ;
#11909=CIRCLE ( 'NONE', #17241, 0.8366141732283465249 ) ;
#11958=CARTESIAN_POINT ( 'NONE',  ( -0.1574803149606299191, 0.07021257666614952320, -0.1553045758542780375 ) ) ;
#11975=LINE ( 'NONE', #1383, #16910 ) ;
#11982=ORIENTED_EDGE ( 'NONE', *, *, #33305, .T. ) ;
#12032=ADVANCED_FACE ( 'NONE', ( #44545 ), #40942, .T. ) ;
#12033=ADVANCED_FACE ( 'NONE', ( #5023 ), #45762, .T. ) ;
#12050=CARTESIAN_POINT ( 'NONE',  ( 0.1476377952755906220, 0.06415291647593752977, -0.1630605872086748620 ) ) ;
#12077=ORIENTED_EDGE ( 'NONE', *, *, #31779, .T. ) ;
#12085=DIRECTION ( 'NONE',  ( 0.000000000000000000, 0.7880107536067203489, -0.6156614753256604011 ) ) ;
#12093=CARTESIAN_POINT ( 'NONE',  ( -0.1574803149606299191, 0.7443365962042343131, -3.523993443072799270 ) ) ;
#12104=DIRECTION ( 'NONE',  ( 0.000000000000000000, -0.7880107536067206819, 0.6156614753256597350 ) ) ;
#12130=ORIENTED_EDGE ( 'NONE', *, *, #30668, .T. ) ;
#12160=DIRECTION ( 'NONE',  ( 0.000000000000000000, 0.000000000000000000, 1.000000000000000000 ) ) ;
#12171=CIRCLE ( 'NONE', #13691, 0.01968503937007870172 ) ;
#12191=DIRECTION ( 'NONE',  ( -1.000000000000000000, -0.000000000000000000, 0.000000000000000000 ) ) ;
#12211=VERTEX_POINT ( 'NONE', #2360 ) ;
#12256=CARTESIAN_POINT ( 'NONE',  ( -0.1476377952755905387, -0.2142072668875215635, -1.269802121763611291 ) ) ;
#12266=DIRECTION ( 'NONE',  ( 6.938893903907227392E-16, -0.6156614753256598460, -0.7880107536067207930 ) ) ;
#12277=ORIENTED_EDGE ( 'NONE', *, *, #40328, .T. ) ;
#12288=ORIENTED_EDGE ( 'NONE', *, *, #16824, .T. ) ;
#12295=EDGE_CURVE ( 'NONE', #19153, #2867, #19779, .T. ) ;
#12303=ORIENTED_EDGE ( 'NONE', *, *, #21297, .T. ) ;
#12340=AXIS2_PLACEMENT_3D ( 'NONE', #27019, #12635, #14858 ) ;
#12377=CARTESIAN_POINT ( 'NONE',  ( -0.1574803149606299191, 0.2876548164643190630, -0.2627373885913885099 ) ) ;
#12382=VECTOR ( 'NONE', #14265, 39.37007874015748143 ) ;
#12423=EDGE_CURVE ( 'NONE', #8964, #8992, #34168, .T. ) ;
#12434=DIRECTION ( 'NONE',  ( 0.000000000000000000, -0.7880107536067207930, 0.6156614753256598460 ) ) ;
#12450=FACE_OUTER_BOUND ( 'NONE', #8035, .T. ) ;
#12477=VERTEX_POINT ( 'NONE', #30244 ) ;
#12484=TOROIDAL_SURFACE ( 'NONE', #34667, 0.7972440944881888925, 0.009842519685039369942 ) ;
#12502=( NAMED_UNIT ( * ) SI_UNIT ( $, .STERADIAN. ) SOLID_ANGLE_UNIT ( ) ) ;
#12524=VERTEX_POINT ( 'NONE', #8383 ) ;
#12533=CARTESIAN_POINT ( 'NONE',  ( -0.2066929133858267931, -0.5175744617845221551, -0.9076376772307637175 ) ) ;
#12541=CARTESIAN_POINT ( 'NONE',  ( -0.1476377952755905387, 0.2512968553230415791, -0.3092734567177705673 ) ) ;
#12635=DIRECTION ( 'NONE',  ( 0.000000000000000000, -0.2432573283306646017, 0.9699617890481188054 ) ) ;
#12660=ORIENTED_EDGE ( 'NONE', *, *, #33754, .T. ) ;
#12675=CARTESIAN_POINT ( 'NONE',  ( -0.2066929133858267931, 0.7443365962042343131, -3.523993443072799270 ) ) ;
#12680=AXIS2_PLACEMENT_3D ( 'NONE', #15297, #34001, #22954 ) ;
#12691=ORIENTED_EDGE ( 'NONE', *, *, #7315, .F. ) ;
#12800=CARTESIAN_POINT ( 'NONE',  ( 0.1574803149606300023, 0.7443365962042343131, -3.523993443072799270 ) ) ;
#12840=DIRECTION ( 'NONE',  ( 0.000000000000000000, 0.2126700594527823618, -0.9771240687918550938 ) ) ;
#12893=LINE ( 'NONE', #27527, #25957 ) ;
#12923=FACE_OUTER_BOUND ( 'NONE', #3972, .T. ) ;
#12924=CYLINDRICAL_SURFACE ( 'NONE', #28574, 0.7381889763779526659 ) ;
#12958=ORIENTED_EDGE ( 'NONE', *, *, #40129, .T. ) ;
#12959=VECTOR ( 'NONE', #13099, 39.37007874015748854 ) ;
#12968=AXIS2_PLACEMENT_3D ( 'NONE', #14509, #29171, #32977 ) ;
#13004=EDGE_CURVE ( 'NONE', #18185, #22505, #35529, .T. ) ;
#13025=DIMENSIONAL_EXPONENTS ( 1.000000000000000000, 0.000000000000000000, 0.000000000000000000, 0.000000000000000000, 0.000000000000000000, 0.000000000000000000, 0.000000000000000000 ) ;
#13075=AXIS2_PLACEMENT_3D ( 'NONE', #40813, #33691, #12104 ) ;
#13077=EDGE_CURVE ( 'NONE', #2020, #47303, #11418, .T. ) ;
#13099=DIRECTION ( 'NONE',  ( -0.000000000000000000, 0.2432573283306645462, -0.9699617890481188054 ) ) ;
#13177=ADVANCED_FACE ( 'NONE', ( #38272 ), #20056, .T. ) ;
#13186=EDGE_CURVE ( 'NONE', #28190, #34488, #39672, .T. ) ;
#13227=ADVANCED_FACE ( 'NONE', ( #45442 ), #7570, .F. ) ;
#13229=FACE_OUTER_BOUND ( 'NONE', #38520, .T. ) ;
#13233=EDGE_CURVE ( 'NONE', #39665, #25724, #8560, .T. ) ;
#13271=DIRECTION ( 'NONE',  ( -1.000000000000000000, -0.000000000000000000, -0.000000000000000000 ) ) ;
#13280=EDGE_CURVE ( 'NONE', #9478, #16549, #12893, .T. ) ;
#13291=EDGE_CURVE ( 'NONE', #46402, #25724, #12171, .T. ) ;
#13327=DIRECTION ( 'NONE',  ( 0.000000000000000000, 0.9699617890481186944, 0.2432573283306648515 ) ) ;
#13382=CARTESIAN_POINT ( 'NONE',  ( -0.1574803149606299191, -0.2274162997038020051, -0.9219983537151217323 ) ) ;
#13397=EDGE_CURVE ( 'NONE', #26907, #19153, #45920, .T. ) ;
#13442=AXIS2_PLACEMENT_3D ( 'NONE', #11448, #23178, #12160 ) ;
#13578=EDGE_LOOP ( 'NONE', ( #25067, #13785, #37749, #44152 ) ) ;
#13582=ADVANCED_FACE ( 'NONE', ( #33243 ), #14535, .T. ) ;
#13586=AXIS2_PLACEMENT_3D ( 'NONE', #23369, #4896, #41772 ) ;
#13588=DIRECTION ( 'NONE',  ( -1.000000000000000000, -0.000000000000000000, 0.000000000000000000 ) ) ;
#13641=ORIENTED_EDGE ( 'NONE', *, *, #18348, .T. ) ;
#13681=DIRECTION ( 'NONE',  ( 0.000000000000000000, 0.000000000000000000, 1.000000000000000000 ) ) ;
#13691=AXIS2_PLACEMENT_3D ( 'NONE', #19345, #30415, #44964 ) ;
#13718=CARTESIAN_POINT ( 'NONE',  ( 0.1968503937007874682, 0.06245656531175267784, -0.1492449156640648367 ) ) ;
#13762=AXIS2_PLACEMENT_3D ( 'NONE', #39549, #6722, #14171 ) ;
#13765=APPLICATION_CONTEXT ( 'automotive_design' ) ;
#13785=ORIENTED_EDGE ( 'NONE', *, *, #38260, .F. ) ;
#13814=DIRECTION ( 'NONE',  ( 1.000000000000000000, 0.000000000000000000, 0.000000000000000000 ) ) ;
#13846=CARTESIAN_POINT ( 'NONE',  ( 0.1476377952755906220, -0.4950321721878526704, -0.8627979602685659222 ) ) ;
#13887=VECTOR ( 'NONE', #12085, 39.37007874015748143 ) ;
#13895=CARTESIAN_POINT ( 'NONE',  ( -0.1574803149606299191, 0.3743908788525359688, -3.616772362661643481 ) ) ;
#13898=FACE_OUTER_BOUND ( 'NONE', #33571, .T. ) ;
#13908=DIRECTION ( 'NONE',  ( 0.000000000000000000, 0.7880107536067184615, -0.6156614753256628436 ) ) ;
#13951=VECTOR ( 'NONE', #43968, 39.37007874015748143 ) ;
#13975=ORIENTED_EDGE ( 'NONE', *, *, #29207, .T. ) ;
#13994=ORIENTED_EDGE ( 'NONE', *, *, #13077, .F. ) ;
#14081=FACE_OUTER_BOUND ( 'NONE', #45253, .T. ) ;
#14128=ORIENTED_EDGE ( 'NONE', *, *, #18243, .F. ) ;
#14171=DIRECTION ( 'NONE',  ( 0.000000000000000000, 0.000000000000000000, 1.000000000000000000 ) ) ;
#14186=EDGE_CURVE ( 'NONE', #24192, #2855, #17556, .T. ) ;
#14197=EDGE_CURVE ( 'NONE', #16549, #22505, #32942, .T. ) ;
#14209=LINE ( 'NONE', #35546, #31575 ) ;
#14265=DIRECTION ( 'NONE',  ( -1.000000000000000000, -0.000000000000000000, -0.000000000000000000 ) ) ;
#14324=DIRECTION ( 'NONE',  ( -1.000000000000000000, -0.000000000000000000, 0.000000000000000000 ) ) ;
#14367=ORIENTED_EDGE ( 'NONE', *, *, #7307, .T. ) ;
#14378=ORIENTED_EDGE ( 'NONE', *, *, #29447, .T. ) ;
#14392=VECTOR ( 'NONE', #30974, 39.37007874015748143 ) ;
#14414=CYLINDRICAL_SURFACE ( 'NONE', #1916, 0.009842519685039423719 ) ;
#14443=CARTESIAN_POINT ( 'NONE',  ( 0.1476377952755906220, 0.5323553679591568333, -0.7566348232351032266 ) ) ;
#14480=VERTEX_POINT ( 'NONE', #23315 ) ;
#14509=CARTESIAN_POINT ( 'NONE',  ( 0.1574803149606300023, 0.4814845645395590679, -0.4766254685646189593 ) ) ;
#14526=EDGE_LOOP ( 'NONE', ( #37633, #3262, #14367, #1765 ) ) ;
#14530=EDGE_CURVE ( 'NONE', #12477, #21515, #29069, .T. ) ;
#14535=CYLINDRICAL_SURFACE ( 'NONE', #24413, 0.009842519685039378616 ) ;
#14580=VECTOR ( 'NONE', #13271, 39.37007874015748143 ) ;
#14676=DIRECTION ( 'NONE',  ( -1.000000000000000000, -0.000000000000000000, 0.000000000000000000 ) ) ;
#14679=EDGE_CURVE ( 'NONE', #5180, #14871, #21418, .T. ) ;
#14685=CIRCLE ( 'NONE', #900, 0.7874015748031495399 ) ;
#14762=EDGE_LOOP ( 'NONE', ( #31881, #830, #46617, #47123, #42697, #19699, #10699, #45335 ) ) ;
#14767=CIRCLE ( 'NONE', #17040, 0.009842519685039387289 ) ;
#14800=FACE_OUTER_BOUND ( 'NONE', #15484, .T. ) ;
#14828=FACE_OUTER_BOUND ( 'NONE', #20789, .T. ) ;
#14858=DIRECTION ( 'NONE',  ( 0.000000000000000000, -0.9699617890481199156, -0.2432573283306598000 ) ) ;
#14860=ORIENTED_EDGE ( 'NONE', *, *, #2783, .T. ) ;
#14871=VERTEX_POINT ( 'NONE', #24311 ) ;
#14887=CARTESIAN_POINT ( 'NONE',  ( 0.1574803149606299746, -0.4410959923581754816, -0.9673892061308019263 ) ) ;
#14911=DIRECTION ( 'NONE',  ( 0.000000000000000000, -0.7880107536067207930, 0.6156614753256598460 ) ) ;
#15017=CIRCLE ( 'NONE', #428, 0.009842519685039399432 ) ;
#15057=FACE_OUTER_BOUND ( 'NONE', #42561, .T. ) ;
#15084=AXIS2_PLACEMENT_3D ( 'NONE', #12541, #22591, #27162 ) ;
#15104=LINE ( 'NONE', #33561, #8809 ) ;
#15112=ORIENTED_EDGE ( 'NONE', *, *, #24241, .F. ) ;
#15123=DIRECTION ( 'NONE',  ( 0.000000000000000000, -0.7880107536067207930, 0.6156614753256598460 ) ) ;
#15164=DIRECTION ( 'NONE',  ( -0.000000000000000000, 0.6156614753256597350, 0.7880107536067206819 ) ) ;
#15230=VERTEX_POINT ( 'NONE', #9866 ) ;
#15245=ORIENTED_EDGE ( 'NONE', *, *, #32097, .F. ) ;
#15256=AXIS2_PLACEMENT_3D ( 'NONE', #25621, #33057, #7852 ) ;
#15263=CARTESIAN_POINT ( 'NONE',  ( 0.1476377952755906220, 0.2573565155132549465, -0.3015174453633734930 ) ) ;
#15297=CARTESIAN_POINT ( 'NONE',  ( -0.1574803149606299191, 1.126631386849005212, -3.440787370833235492 ) ) ;
#15308=AXIS2_PLACEMENT_3D ( 'NONE', #21585, #36226, #40947 ) ;
#15342=ORIENTED_EDGE ( 'NONE', *, *, #35660, .F. ) ;
#15360=CARTESIAN_POINT ( 'NONE',  ( 0.2066929133858268486, -0.3022687907404924545, -1.075852903322848331 ) ) ;
#15382=EDGE_CURVE ( 'NONE', #6831, #28708, #27159, .T. ) ;
#15399=DIRECTION ( 'NONE',  ( 0.000000000000000000, -0.6156614753256497430, -0.7880107536067285645 ) ) ;
#15413=VECTOR ( 'NONE', #41811, 39.37007874015748143 ) ;
#15417=EDGE_LOOP ( 'NONE', ( #17471, #10465, #45672, #45932 ) ) ;
#15433=EDGE_CURVE ( 'NONE', #5246, #12477, #40013, .T. ) ;
#15437=DIRECTION ( 'NONE',  ( -1.000000000000000000, -0.000000000000000000, 0.000000000000000000 ) ) ;
#15454=CARTESIAN_POINT ( 'NONE',  ( 0.1968503937007874682, 0.07021257666614930115, -0.1553045758542778432 ) ) ;
#15461=DIRECTION ( 'NONE',  ( 0.000000000000000000, -0.7880107536067181284, 0.6156614753256632877 ) ) ;
#15467=EDGE_LOOP ( 'NONE', ( #35076, #2485, #481, #20634 ) ) ;
#15484=EDGE_LOOP ( 'NONE', ( #5420, #33361, #16884, #26578 ) ) ;
#15486=VECTOR ( 'NONE', #971, 39.37007874015748143 ) ;
#15535=ORIENTED_EDGE ( 'NONE', *, *, #19757, .T. ) ;
#15554=ADVANCED_FACE ( 'NONE', ( #43616 ), #34438, .F. ) ;
#15573=CARTESIAN_POINT ( 'NONE',  ( 0.1476377952755906220, 0.3743908788525356912, -3.616772362661642148 ) ) ;
#15612=EDGE_CURVE ( 'NONE', #11278, #43605, #35967, .T. ) ;
#15628=CARTESIAN_POINT ( 'NONE',  ( -0.1574803149606299191, 0.5257908685547681982, -0.4487896632427120225 ) ) ;
#15688=CARTESIAN_POINT ( 'NONE',  ( 0.1476377952755906220, 1.117014023967195735, -3.442880580079816788 ) ) ;
#15691=AXIS2_PLACEMENT_3D ( 'NONE', #36128, #29226, #145 ) ;
#15702=FACE_OUTER_BOUND ( 'NONE', #22126, .T. ) ;
#15737=AXIS2_PLACEMENT_3D ( 'NONE', #29450, #136, #11427 ) ;
#15756=CARTESIAN_POINT ( 'NONE',  ( -0.2066929133858267931, 0.04819563354825918966, -0.1381030546566545669 ) ) ;
#15789=CYLINDRICAL_SURFACE ( 'NONE', #12680, 0.04921259842519678379 ) ;
#15805=CARTESIAN_POINT ( 'NONE',  ( 0.1476377952755906220, -0.9875035750853327077, -1.463737590216208861 ) ) ;
#15807=ORIENTED_EDGE ( 'NONE', *, *, #34172, .F. ) ;
#15871=VECTOR ( 'NONE', #41724, 39.37007874015748143 ) ;
#15909=VECTOR ( 'NONE', #8476, 39.37007874015748143 ) ;
#15971=APPLICATION_CONTEXT ( 'automotive_design' ) ;
#16009=TOROIDAL_SURFACE ( 'NONE', #37386, 0.7874015748031496509, 0.04921259842519685318 ) ;
#16020=DIRECTION ( 'NONE',  ( 0.000000000000000000, -0.7880107536067207930, 0.6156614753256598460 ) ) ;
#16039=ORIENTED_EDGE ( 'NONE', *, *, #30319, .T. ) ;
#16042=DIRECTION ( 'NONE',  ( 1.000000000000000000, 0.000000000000000000, 0.000000000000000000 ) ) ;
#16101=LINE ( 'NONE', #18949, #42270 ) ;
#16104=EDGE_LOOP ( 'NONE', ( #3113, #8682, #20150, #21932 ) ) ;
#16107=CARTESIAN_POINT ( 'NONE',  ( 0.1574803149606299746, 0.5900595452500136950, -0.7440755677556079029 ) ) ;
#16143=ADVANCED_FACE ( 'NONE', ( #33996 ), #32179, .T. ) ;
#16223=CARTESIAN_POINT ( 'NONE',  ( -0.2066929133858267931, 0.5900595452500136950, -0.7440755677556079029 ) ) ;
#16238=AXIS2_PLACEMENT_3D ( 'NONE', #26114, #4499, #19134 ) ;
#16253=CARTESIAN_POINT ( 'NONE',  ( -0.1574803149606299191, 0.08669520607260540468, -0.1182208702464774136 ) ) ;
#16272=DIRECTION ( 'NONE',  ( 0.000000000000000000, 0.000000000000000000, 1.000000000000000000 ) ) ;
#16274=AXIS2_PLACEMENT_3D ( 'NONE', #46784, #10147, #39591 ) ;
#16275=DIRECTION ( 'NONE',  ( 0.000000000000000000, -0.7880107536067207930, 0.6156614753256598460 ) ) ;
#16300=ORIENTED_EDGE ( 'NONE', *, *, #5750, .F. ) ;
#16321=ORIENTED_EDGE ( 'NONE', *, *, #45438, .T. ) ;
#16358=ADVANCED_FACE ( 'NONE', ( #2079 ), #30412, .F. ) ;
#16360=EDGE_LOOP ( 'NONE', ( #12277, #45868, #39608, #39557 ) ) ;
#16449=LINE ( 'NONE', #35368, #12959 ) ;
#16461=DIRECTION ( 'NONE',  ( 0.000000000000000000, -0.2126700594528006805, 0.9771240687918512080 ) ) ;
#16481=DIRECTION ( 'NONE',  ( 0.000000000000000000, 0.000000000000000000, 1.000000000000000000 ) ) ;
#16495=FACE_OUTER_BOUND ( 'NONE', #28689, .T. ) ;
#16532=ORIENTED_EDGE ( 'NONE', *, *, #37986, .F. ) ;
#16549=VERTEX_POINT ( 'NONE', #20234 ) ;
#16554=DIRECTION ( 'NONE',  ( 0.000000000000000000, -0.6156614753256597350, -0.7880107536067207930 ) ) ;
#16572=ORIENTED_EDGE ( 'NONE', *, *, #9036, .F. ) ;
#16588=EDGE_LOOP ( 'NONE', ( #22013, #23169, #44740, #11334 ) ) ;
#16624=CARTESIAN_POINT ( 'NONE',  ( -0.1574803149606299191, 0.5900595452500136950, -0.7440755677556079029 ) ) ;
#16637=ORIENTED_EDGE ( 'NONE', *, *, #35297, .T. ) ;
#16672=VECTOR ( 'NONE', #29405, 39.37007874015748143 ) ;
#16685=LINE ( 'NONE', #37532, #16741 ) ;
#16691=ORIENTED_EDGE ( 'NONE', *, *, #36095, .F. ) ;
#16707=AXIS2_PLACEMENT_3D ( 'NONE', #33553, #670, #2108 ) ;
#16712=DIRECTION ( 'NONE',  ( 1.000000000000000000, 0.000000000000000000, 0.000000000000000000 ) ) ;
#16741=VECTOR ( 'NONE', #30388, 39.37007874015748143 ) ;
#16821=ADVANCED_FACE ( 'NONE', ( #11632 ), #30566, .T. ) ;
#16824=EDGE_CURVE ( 'NONE', #2521, #6124, #32841, .T. ) ;
#16868=ORIENTED_EDGE ( 'NONE', *, *, #37161, .T. ) ;
#16884=ORIENTED_EDGE ( 'NONE', *, *, #15612, .F. ) ;
#16894=VECTOR ( 'NONE', #30390, 39.37007874015748854 ) ;
#16910=VECTOR ( 'NONE', #442, 39.37007874015748854 ) ;
#16949=CARTESIAN_POINT ( 'NONE',  ( -0.1476377952755905387, 0.07021257666615011994, -0.1553045758542774268 ) ) ;
#16972=CARTESIAN_POINT ( 'NONE',  ( 0.1574803149606300023, 2.123129472280982366, -1.759219038810944324 ) ) ;
#16994=EDGE_CURVE ( 'NONE', #17869, #26907, #32986, .T. ) ;
#17025=CARTESIAN_POINT ( 'NONE',  ( 0.1476377952755906220, -0.9875035750853327077, -1.463737590216208861 ) ) ;
#17040=AXIS2_PLACEMENT_3D ( 'NONE', #40111, #29866, #22382 ) ;
#17113=ADVANCED_FACE ( 'NONE', ( #41517 ), #34379, .F. ) ;
#17148=AXIS2_PLACEMENT_3D ( 'NONE', #31181, #42400, #3090 ) ;
#17164=ORIENTED_EDGE ( 'NONE', *, *, #22775, .F. ) ;
#17201=CYLINDRICAL_SURFACE ( 'NONE', #15691, 0.009842519685039371677 ) ;
#17241=AXIS2_PLACEMENT_3D ( 'NONE', #30220, #18905, #45245 ) ;
#17372=CYLINDRICAL_SURFACE ( 'NONE', #19973, 0.009842519685039274532 ) ;
#17380=ORIENTED_EDGE ( 'NONE', *, *, #38350, .F. ) ;
#17400=CARTESIAN_POINT ( 'NONE',  ( -0.2066929133858267931, 0.3171096708378827178, -3.631137952917390166 ) ) ;
#17409=CARTESIAN_POINT ( 'NONE',  ( -0.1574803149606299191, 1.174718201258053485, -3.430321324600322352 ) ) ;
#17471=ORIENTED_EDGE ( 'NONE', *, *, #14530, .T. ) ;
#17520=EDGE_CURVE ( 'NONE', #14480, #8597, #21522, .T. ) ;
#17543=CIRCLE ( 'NONE', #38983, 0.3912448816427701037 ) ;
#17556=CIRCLE ( 'NONE', #31334, 0.04921259842519688094 ) ;
#17687=ORIENTED_EDGE ( 'NONE', *, *, #29207, .F. ) ;
#17739=ORIENTED_EDGE ( 'NONE', *, *, #46961, .T. ) ;
#17763=AXIS2_PLACEMENT_3D ( 'NONE', #28912, #43476, #41047 ) ;
#17869=VERTEX_POINT ( 'NONE', #21554 ) ;
#17877=VERTEX_POINT ( 'NONE', #13895 ) ;
#17917=EDGE_CURVE ( 'NONE', #12524, #47303, #32253, .T. ) ;
#17993=DIRECTION ( 'NONE',  ( 0.000000000000000000, 0.2432573283306646017, -0.9699617890481188054 ) ) ;
#17994=VECTOR ( 'NONE', #28709, 39.37007874015748143 ) ;
#18051=ORIENTED_EDGE ( 'NONE', *, *, #11008, .F. ) ;
#18063=AXIS2_PLACEMENT_3D ( 'NONE', #43091, #10295, #42614 ) ;
#18081=ADVANCED_FACE ( 'NONE', ( #26109 ), #8350, .F. ) ;
#18170=CARTESIAN_POINT ( 'NONE',  ( -0.1476377952755905387, -0.4075443641102559078, -0.9311509272141712534 ) ) ;
#18184=EDGE_CURVE ( 'NONE', #39665, #39149, #4655, .T. ) ;
#18185=VERTEX_POINT ( 'NONE', #22254 ) ;
#18230=DIRECTION ( 'NONE',  ( 1.000000000000000000, 0.000000000000000000, 0.000000000000000000 ) ) ;
#18239=EDGE_CURVE ( 'NONE', #2020, #7195, #11975, .T. ) ;
#18240=CIRCLE ( 'NONE', #16707, 0.7874015748031496509 ) ;
#18243=EDGE_CURVE ( 'NONE', #28708, #45599, #34532, .T. ) ;
#18248=DIRECTION ( 'NONE',  ( 4.272009658007763174E-15, -0.6156614753256599570, -0.7880107536067207930 ) ) ;
#18256=DIRECTION ( 'NONE',  ( -0.000000000000000000, 0.9771240687918548717, 0.2126700594527834720 ) ) ;
#18259=CARTESIAN_POINT ( 'NONE',  ( 0.1574803149606300023, 0.06245656531175268478, -0.1492449156640648089 ) ) ;
#18304=CARTESIAN_POINT ( 'NONE',  ( -0.1574803149606299191, 0.5323553679591567223, -0.7566348232351032266 ) ) ;
#18309=CARTESIAN_POINT ( 'NONE',  ( 0.1574803149606299746, -0.9875035750853327077, -1.463737590216208861 ) ) ;
#18325=CARTESIAN_POINT ( 'NONE',  ( 0.1574803149606300023, 1.126631386849004990, -3.440787370833234160 ) ) ;
#18326=LINE ( 'NONE', #85, #16672 ) ;
#18348=EDGE_CURVE ( 'NONE', #12211, #25679, #44454, .T. ) ;
#18356=EDGE_CURVE ( 'NONE', #20344, #39970, #5376, .T. ) ;
#18359=DIRECTION ( 'NONE',  ( 1.000000000000000000, 0.000000000000000000, 0.000000000000000000 ) ) ;
#18397=CARTESIAN_POINT ( 'NONE',  ( -0.1574803149606299191, 0.4954925676037022497, -0.4875697200146963950 ) ) ;
#18478=DIRECTION ( 'NONE',  ( 0.000000000000000000, 0.7880107536067203489, -0.6156614753256602901 ) ) ;
#18505=AXIS2_PLACEMENT_3D ( 'NONE', #36386, #46901, #6409 ) ;
#18545=CARTESIAN_POINT ( 'NONE',  ( 0.1476377952755906220, -0.4812165006432430059, -0.8611016091043821596 ) ) ;
#18576=PRESENTATION_STYLE_ASSIGNMENT (( #30747 ) ) ;
#18604=VECTOR ( 'NONE', #18863, 39.37007874015748854 ) ;
#18620=CARTESIAN_POINT ( 'NONE',  ( 0.2066929133858268486, -0.2237541348899642901, -1.272196386806234925 ) ) ;
#18664=DIRECTION ( 'NONE',  ( 4.272009658007748186E-16, 0.7880107536067211260, -0.6156614753256594019 ) ) ;
#18667=ORIENTED_EDGE ( 'NONE', *, *, #34172, .T. ) ;
#18692=DIRECTION ( 'NONE',  ( 0.000000000000000000, 0.7880107536067184615, -0.6156614753256628436 ) ) ;
#18700=AXIS2_PLACEMENT_3D ( 'NONE', #18325, #25766, #40336 ) ;
#18701=EDGE_CURVE ( 'NONE', #22505, #33099, #29689, .T. ) ;
#18705=EDGE_CURVE ( 'NONE', #7195, #23068, #30020, .T. ) ;
#18720=DIRECTION ( 'NONE',  ( 0.000000000000000000, -0.6156614753256604011, -0.7880107536067203489 ) ) ;
#18731=LINE ( 'NONE', #507, #11688 ) ;
#18769=AXIS2_PLACEMENT_3D ( 'NONE', #32588, #29494, #44038 ) ;
#18786=DIRECTION ( 'NONE',  ( -0.000000000000000000, 0.2432573283306645462, -0.9699617890481188054 ) ) ;
#18794=ORIENTED_EDGE ( 'NONE', *, *, #15433, .T. ) ;
#18809=EDGE_LOOP ( 'NONE', ( #3232, #1453, #32864, #5140 ) ) ;
#18827=DIRECTION ( 'NONE',  ( 1.000000000000000000, 0.000000000000000000, 0.000000000000000000 ) ) ;
#18863=DIRECTION ( 'NONE',  ( -0.000000000000000000, -0.2126700594527834443, 0.9771240687918547607 ) ) ;
#18888=DIRECTION ( 'NONE',  ( 0.000000000000000000, 0.2126700594527834443, -0.9771240687918547607 ) ) ;
#18905=DIRECTION ( 'NONE',  ( -1.000000000000000000, -0.000000000000000000, 0.000000000000000000 ) ) ;
#18929=CARTESIAN_POINT ( 'NONE',  ( 0.1805937969716511771, -0.4173683960833115547, -0.9859272360519073519 ) ) ;
#18949=CARTESIAN_POINT ( 'NONE',  ( -0.1574803149606299191, -0.5010918323780659822, -0.8705539716229625524 ) ) ;
#18965=ORIENTED_EDGE ( 'NONE', *, *, #8699, .T. ) ;
#19012=CARTESIAN_POINT ( 'NONE',  ( 0.1476377952755906220, -0.2237541348899636795, -1.272196386806235813 ) ) ;
#19040=LENGTH_MEASURE_WITH_UNIT ( LENGTH_MEASURE( 0.02539999999999999897 ), #34557 ) ;
#19057=VECTOR ( 'NONE', #36040, 39.37007874015748143 ) ;
#19078=DIRECTION ( 'NONE',  ( 0.000000000000000000, -0.7880107536067233465, 0.6156614753256566264 ) ) ;
#19090=DIRECTION ( 'NONE',  ( 0.000000000000000000, -0.6156614753256596240, -0.7880107536067210150 ) ) ;
#19134=DIRECTION ( 'NONE',  ( 0.000000000000000000, -0.6156614753256597350, -0.7880107536067207930 ) ) ;
#19148=EDGE_CURVE ( 'NONE', #21515, #44611, #46360, .T. ) ;
#19153=VERTEX_POINT ( 'NONE', #31778 ) ;
#19194=AXIS2_PLACEMENT_3D ( 'NONE', #43306, #21027, #6650 ) ;
#19215=CARTESIAN_POINT ( 'NONE',  ( -0.1574803149606299191, 0.5419727308409657551, -0.7545416139885203766 ) ) ;
#19239=CARTESIAN_POINT ( 'NONE',  ( -0.1476377952755905387, 1.126631386849005878, -3.440787370833236380 ) ) ;
#19252=DIRECTION ( 'NONE',  ( 0.000000000000000000, 0.2126700594527834720, -0.9771240687918549828 ) ) ;
#19279=DIRECTION ( 'NONE',  ( -1.000000000000000000, 0.000000000000000000, 0.000000000000000000 ) ) ;
#19299=AXIS2_PLACEMENT_3D ( 'NONE', #10357, #31928, #46517 ) ;
#19320=DIRECTION ( 'NONE',  ( 0.000000000000000000, 0.6156614753256602901, 0.7880107536067203489 ) ) ;
#19322=CIRCLE ( 'NONE', #46101, 0.009842519685039371677 ) ;
#19345=CARTESIAN_POINT ( 'NONE',  ( 0.1476377952755906220, -0.4889725119976396916, -0.8550419489141691809 ) ) ;
#19426=DIRECTION ( 'NONE',  ( 1.000000000000000000, 0.000000000000000000, -0.000000000000000000 ) ) ;
#19442=ORIENTED_EDGE ( 'NONE', *, *, #23008, .F. ) ;
#19460=CIRCLE ( 'NONE', #5717, 0.009842519685039399432 ) ;
#19505=DIRECTION ( 'NONE',  ( 0.000000000000000000, 5.311252123978373147E-15, 1.000000000000000000 ) ) ;
#19526=EDGE_LOOP ( 'NONE', ( #34644, #9810, #46323, #16868 ) ) ;
#19530=CIRCLE ( 'NONE', #18769, 0.009842519685039378616 ) ;
#19537=AXIS2_PLACEMENT_3D ( 'NONE', #46175, #3025, #35416 ) ;
#19586=DIRECTION ( 'NONE',  ( 0.000000000000000000, -0.2126700594527834720, 0.9771240687918549828 ) ) ;
#19599=AXIS2_PLACEMENT_3D ( 'NONE', #3635, #18256, #6990 ) ;
#19613=CARTESIAN_POINT ( 'NONE',  ( 0.1673228346456693827, 0.06415291647593675262, -0.1630605872086743346 ) ) ;
#19624=ORIENTED_EDGE ( 'NONE', *, *, #13291, .T. ) ;
#19686=DIRECTION ( 'NONE',  ( 0.000000000000000000, 0.2126700594527830002, -0.9771240687918550938 ) ) ;
#19699=ORIENTED_EDGE ( 'NONE', *, *, #45386, .T. ) ;
#19719=EDGE_CURVE ( 'NONE', #6124, #8964, #41156, .T. ) ;
#19757=EDGE_CURVE ( 'NONE', #6624, #12524, #28393, .T. ) ;
#19779=CIRCLE ( 'NONE', #34343, 0.04921259842519683236 ) ;
#19844=DIRECTION ( 'NONE',  ( -0.000000000000000000, 0.2126700594527834443, -0.9771240687918547607 ) ) ;
#19948=CARTESIAN_POINT ( 'NONE',  ( 0.2066929133858268486, 1.126631386849005212, -3.440787370833234604 ) ) ;
#19973=AXIS2_PLACEMENT_3D ( 'NONE', #24118, #32009, #46601 ) ;
#19992=AXIS2_PLACEMENT_3D ( 'NONE', #1280, #4879, #19505 ) ;
#20002=EDGE_LOOP ( 'NONE', ( #20875, #36175, #11225, #31063 ) ) ;
#20011=ORIENTED_EDGE ( 'NONE', *, *, #31414, .T. ) ;
#20012=AXIS2_PLACEMENT_3D ( 'NONE', #5219, #20320, #23687 ) ;
#20056=PLANE ( 'NONE',  #28255 ) ;
#20071=FACE_OUTER_BOUND ( 'NONE', #1652, .T. ) ;
#20111=CARTESIAN_POINT ( 'NONE',  ( 0.1574803149606299746, 0.3648440108500936585, -3.619166627704266670 ) ) ;
#20150=ORIENTED_EDGE ( 'NONE', *, *, #22835, .F. ) ;
#20224=ORIENTED_EDGE ( 'NONE', *, *, #12295, .T. ) ;
#20234=CARTESIAN_POINT ( 'NONE',  ( -0.1968503937007874127, -0.5192708129487058066, -0.8938220056861535534 ) ) ;
#20304=VECTOR ( 'NONE', #45003, 39.37007874015748143 ) ;
#20320=DIRECTION ( 'NONE',  ( 1.000000000000000000, 0.000000000000000000, -0.000000000000000000 ) ) ;
#20344=VERTEX_POINT ( 'NONE', #9733 ) ;
#20350=AXIS2_PLACEMENT_3D ( 'NONE', #23421, #16461, #6117 ) ;
#20388=CARTESIAN_POINT ( 'NONE',  ( -0.1574803149606299191, -0.9875035750853327077, -1.463737590216208861 ) ) ;
#20399=EDGE_LOOP ( 'NONE', ( #39552, #15807, #39505, #2074 ) ) ;
#20437=CARTESIAN_POINT ( 'NONE',  ( -0.2066929133858267931, 0.2876548164643190630, -0.2627373885913885099 ) ) ;
#20542=CARTESIAN_POINT ( 'NONE',  ( -0.2026160082443592969, -0.5228204797047604213, -0.8983653719476394350 ) ) ;
#20624=DIRECTION ( 'NONE',  ( 0.000000000000000000, 0.000000000000000000, 1.000000000000000000 ) ) ;
#20634=ORIENTED_EDGE ( 'NONE', *, *, #34007, .F. ) ;
#20700=EDGE_LOOP ( 'NONE', ( #29959, #30649, #9520, #10256 ) ) ;
#20789=EDGE_LOOP ( 'NONE', ( #6661, #1779, #39270, #30666 ) ) ;
#20791=FACE_OUTER_BOUND ( 'NONE', #3845, .T. ) ;
#20792=CARTESIAN_POINT ( 'NONE',  ( -0.1476377952755905387, -0.4872761608334559846, -0.8688576204587790119 ) ) ;
#20860=AXIS2_PLACEMENT_3D ( 'NONE', #25692, #32652, #10835 ) ;
#20875=ORIENTED_EDGE ( 'NONE', *, *, #27637, .T. ) ;
#21001=VECTOR ( 'NONE', #24527, 39.37007874015748143 ) ;
#21012=EDGE_LOOP ( 'NONE', ( #14860, #43783, #1407, #2299 ) ) ;
#21027=DIRECTION ( 'NONE',  ( -1.000000000000000000, -0.000000000000000000, 0.000000000000000000 ) ) ;
#21090=EDGE_LOOP ( 'NONE', ( #16637, #700, #24015, #15342 ) ) ;
#21101=DIRECTION ( 'NONE',  ( 0.000000000000000000, -0.2432573283306649070, 0.9699617890481186944 ) ) ;
#21111=MANIFOLD_SOLID_BREP ( 'Link Bar', #39268 ) ;
#21123=CARTESIAN_POINT ( 'NONE',  ( 0.1673228346456693549, -0.4812165006432427838, -0.8611016091043821596 ) ) ;
#21130=EDGE_CURVE ( 'NONE', #46334, #7028, #26157, .T. ) ;
#21134=FACE_OUTER_BOUND ( 'NONE', #29620, .T. ) ;
#21138=CARTESIAN_POINT ( 'NONE',  ( 0.1574803149606300023, -0.2142072668875218133, -1.269802121763611291 ) ) ;
#21297=EDGE_CURVE ( 'NONE', #23068, #25630, #3141, .T. ) ;
#21355=DIRECTION ( 'NONE',  ( 0.000000000000000000, -0.6156614753256598460, -0.7880107536067207930 ) ) ;
#21377=DIRECTION ( 'NONE',  ( 1.000000000000000000, -0.000000000000000000, -0.000000000000000000 ) ) ;
#21410=VECTOR ( 'NONE', #30869, 39.37007874015748143 ) ;
#21418=CIRCLE ( 'NONE', #8389, 0.7874015748031496509 ) ;
#21515=VERTEX_POINT ( 'NONE', #7372 ) ;
#21522=CIRCLE ( 'NONE', #22266, 0.009842519685039354330 ) ;
#21553=ORIENTED_EDGE ( 'NONE', *, *, #9036, .T. ) ;
#21554=CARTESIAN_POINT ( 'NONE',  ( -0.2066929133858267931, 0.3648440108500937140, -3.619166627704267114 ) ) ;
#21585=CARTESIAN_POINT ( 'NONE',  ( 0.1574803149606300023, 1.126631386849004990, -3.440787370833234604 ) ) ;
#21589=ORIENTED_EDGE ( 'NONE', *, *, #44567, .T. ) ;
#21603=EDGE_CURVE ( 'NONE', #14480, #23115, #43057, .T. ) ;
#21643=CARTESIAN_POINT ( 'NONE',  ( 0.1574803149606300023, 0.06851622550196635741, -0.1414889043096673460 ) ) ;
#21704=ORIENTED_EDGE ( 'NONE', *, *, #5256, .T. ) ;
#21777=CIRCLE ( 'NONE', #42387, 0.7874015748031495399 ) ;
#21803=DIRECTION ( 'NONE',  ( 0.000000000000000000, -0.7880107536067207930, 0.6156614753256598460 ) ) ;
#21831=DIRECTION ( 'NONE',  ( 0.000000000000000000, -0.2126700594527834443, 0.9771240687918547607 ) ) ;
#21840=DIRECTION ( 'NONE',  ( 0.000000000000000000, -0.6156614753256598460, -0.7880107536067207930 ) ) ;
#21932=ORIENTED_EDGE ( 'NONE', *, *, #25154, .F. ) ;
#21964=CARTESIAN_POINT ( 'NONE',  ( -0.1476377952755905387, 0.2573565155132548909, -0.3015174453633734930 ) ) ;
#21973=EDGE_CURVE ( 'NONE', #42574, #15230, #38423, .T. ) ;
#22013=ORIENTED_EDGE ( 'NONE', *, *, #17520, .T. ) ;
#22032=CARTESIAN_POINT ( 'NONE',  ( -0.1574803149606299191, -0.2714884749021748145, -1.284167712019358198 ) ) ;
#22033=CYLINDRICAL_SURFACE ( 'NONE', #12340, 0.04921259842519676991 ) ;
#22044=LINE ( 'NONE', #3598, #29844 ) ;
#22069=CARTESIAN_POINT ( 'NONE',  ( -0.1968503937007874127, 0.1005108776172154716, -0.1165245190822937205 ) ) ;
#22111=ORIENTED_EDGE ( 'NONE', *, *, #40129, .F. ) ;
#22126=EDGE_LOOP ( 'NONE', ( #45946, #30891, #4709, #4126 ) ) ;
#22197=DIRECTION ( 'NONE',  ( -0.000000000000000000, 0.6156614753256597350, 0.7880107536067206819 ) ) ;
#22214=EDGE_LOOP ( 'NONE', ( #2375, #25891, #36622, #35348 ) ) ;
#22215=DIRECTION ( 'NONE',  ( 0.000000000000000000, 0.000000000000000000, -1.000000000000000000 ) ) ;
#22247=LINE ( 'NONE', #36421, #29419 ) ;
#22254=CARTESIAN_POINT ( 'NONE',  ( 0.2066929133858268486, -0.5175744617845222662, -0.9076376772307633845 ) ) ;
#22266=AXIS2_PLACEMENT_3D ( 'NONE', #34324, #42177, #45307 ) ;
#22294=CARTESIAN_POINT ( 'NONE',  ( -0.2066929133858267931, -0.2714884749021748145, -1.284167712019358198 ) ) ;
#22298=ORIENTED_EDGE ( 'NONE', *, *, #19148, .F. ) ;
#22299=ORIENTED_EDGE ( 'NONE', *, *, #40328, .F. ) ;
#22382=DIRECTION ( 'NONE',  ( 0.000000000000000000, 0.9699617890481186944, 0.2432573283306645462 ) ) ;
#22391=CARTESIAN_POINT ( 'NONE',  ( -0.1805243946129686250, -0.4175072877304116248, -0.9858187220043870269 ) ) ;
#22401=ORIENTED_EDGE ( 'NONE', *, *, #3254, .T. ) ;
#22414=EDGE_CURVE ( 'NONE', #39665, #45117, #9359, .T. ) ;
#22419=VECTOR ( 'NONE', #18827, 39.37007874015748143 ) ;
#22461=AXIS2_PLACEMENT_3D ( 'NONE', #17025, #1927, #46238 ) ;
#22473=FACE_OUTER_BOUND ( 'NONE', #3901, .T. ) ;
#22498=EDGE_CURVE ( 'NONE', #39149, #42397, #43181, .T. ) ;
#22505=VERTEX_POINT ( 'NONE', #3170 ) ;
#22531=CARTESIAN_POINT ( 'NONE',  ( 0.1647351823960283845, -0.4387500173593407160, -0.9692220826775356235 ) ) ;
#22575=CIRCLE ( 'NONE', #15737, 0.009842519685039378616 ) ;
#22591=DIRECTION ( 'NONE',  ( 0.000000000000000000, 0.7880107536067203489, -0.6156614753256602901 ) ) ;
#22601=ORIENTED_EDGE ( 'NONE', *, *, #34924, .T. ) ;
#22639=CARTESIAN_POINT ( 'NONE',  ( -0.1925018001412950874, -0.3879436464012143704, -1.008916370042088673 ) ) ;
#22642=PLANE ( 'NONE',  #12968 ) ;
#22654=SURFACE_STYLE_FILL_AREA ( #40830 ) ;
#22660=ADVANCED_FACE ( 'NONE', ( #25723 ), #40522, .F. ) ;
#22670=CIRCLE ( 'NONE', #2014, 0.4404574800679669777 ) ;
#22775=EDGE_CURVE ( 'NONE', #30092, #39149, #18731, .T. ) ;
#22835=EDGE_CURVE ( 'NONE', #23380, #5132, #33125, .T. ) ;
#22836=CYLINDRICAL_SURFACE ( 'NONE', #42235, 0.8366141732283466359 ) ;
#22850=AXIS2_PLACEMENT_3D ( 'NONE', #2512, #35601, #13327 ) ;
#22860=EDGE_LOOP ( 'NONE', ( #11159, #9999, #8267, #10275 ) ) ;
#22873=EDGE_LOOP ( 'NONE', ( #15535, #30967, #13994, #38016 ) ) ;
#22906=CARTESIAN_POINT ( 'NONE',  ( -0.2066929133858267931, 0.7443365962042343131, -3.964450923140766303 ) ) ;
#22911=CARTESIAN_POINT ( 'NONE',  ( 0.2066929133858268486, 0.07021257666614924564, -0.1553045758542777877 ) ) ;
#22918=CARTESIAN_POINT ( 'NONE',  ( 0.1476377952755906220, 0.2512968553230415791, -0.3092734567177705673 ) ) ;
#22951=DIRECTION ( 'NONE',  ( 0.000000000000000000, 0.000000000000000000, 1.000000000000000000 ) ) ;
#22954=DIRECTION ( 'NONE',  ( 0.000000000000000000, -0.9771240687918556489, -0.2126700594527800303 ) ) ;
#22973=LINE ( 'NONE', #38061, #27053 ) ;
#22984=DIRECTION ( 'NONE',  ( 0.000000000000000000, 0.000000000000000000, 1.000000000000000000 ) ) ;
#22988=CARTESIAN_POINT ( 'NONE',  ( 0.1574803149606300023, -0.2237541348899639571, -1.272196386806235813 ) ) ;
#23008=EDGE_CURVE ( 'NONE', #34485, #25630, #46070, .T. ) ;
#23020=EDGE_CURVE ( 'NONE', #5132, #12211, #14209, .T. ) ;
#23032=AXIS2_PLACEMENT_3D ( 'NONE', #19613, #29974, #26357 ) ;
#23068=VERTEX_POINT ( 'NONE', #46774 ) ;
#23072=AXIS2_PLACEMENT_3D ( 'NONE', #389, #44230, #30153 ) ;
#23087=VECTOR ( 'NONE', #43537, 39.37007874015748143 ) ;
#23104=FACE_OUTER_BOUND ( 'NONE', #6047, .T. ) ;
#23115=VERTEX_POINT ( 'NONE', #21138 ) ;
#23116=EDGE_CURVE ( 'NONE', #23380, #14480, #10139, .T. ) ;
#23160=CARTESIAN_POINT ( 'NONE',  ( 0.1564141481333313488, -0.4043448265461809243, -0.9276852126764746354 ) ) ;
#23169=ORIENTED_EDGE ( 'NONE', *, *, #28163, .F. ) ;
#23178=DIRECTION ( 'NONE',  ( 1.000000000000000000, 0.000000000000000000, -0.000000000000000000 ) ) ;
#23222=DIRECTION ( 'NONE',  ( 0.000000000000000000, -0.9699617890481251337, -0.2432573283306392609 ) ) ;
#23230=CARTESIAN_POINT ( 'NONE',  ( 0.1574803149606300023, 0.2573565155132531701, -0.3015174453633727714 ) ) ;
#23269=DIRECTION ( 'NONE',  ( 0.000000000000000000, 0.9699617890481186944, 0.2432573283306645462 ) ) ;
#23315=CARTESIAN_POINT ( 'NONE',  ( 0.1574803149606300023, 0.3743908788525358022, -3.616772362661642592 ) ) ;
#23318=ORIENTED_EDGE ( 'NONE', *, *, #45386, .F. ) ;
#23321=CARTESIAN_POINT ( 'NONE',  ( -0.1673228346456692994, 0.05639690512153998359, -0.1570009270184610506 ) ) ;
#23345=AXIS2_PLACEMENT_3D ( 'NONE', #24251, #2418, #13681 ) ;
#23353=ADVANCED_FACE ( 'NONE', ( #20791 ), #24400, .T. ) ;
#23369=CARTESIAN_POINT ( 'NONE',  ( 0.1476377952755906220, -0.4933358210236691854, -0.8766136318131759753 ) ) ;
#23380=VERTEX_POINT ( 'NONE', #5475 ) ;
#23421=CARTESIAN_POINT ( 'NONE',  ( -0.1476377952755905387, 1.117014023967196179, -3.442880580079819008 ) ) ;
#23431=DIRECTION ( 'NONE',  ( -1.000000000000000000, -0.000000000000000000, 0.000000000000000000 ) ) ;
#23530=CIRCLE ( 'NONE', #13586, 0.009842519685039378616 ) ;
#23542=SURFACE_SIDE_STYLE ('',( #22654 ) ) ;
#23557=DIRECTION ( 'NONE',  ( 0.000000000000000000, -0.7880107536067207930, 0.6156614753256598460 ) ) ;
#23588=DIRECTION ( 'NONE',  ( -0.000000000000000000, 0.2126700594527834443, -0.9771240687918547607 ) ) ;
#23614=EDGE_CURVE ( 'NONE', #23115, #7550, #14767, .T. ) ;
#23653=AXIS2_PLACEMENT_3D ( 'NONE', #18259, #14911, #29574 ) ;
#23670=CARTESIAN_POINT ( 'NONE',  ( 0.1476377952755906220, 0.7443365962042343131, -3.523993443072799270 ) ) ;
#23687=DIRECTION ( 'NONE',  ( 0.000000000000000000, -1.778091562876227272E-15, 1.000000000000000000 ) ) ;
#23690=DIRECTION ( 'NONE',  ( 0.000000000000000000, 0.7880107536067203489, -0.6156614753256604011 ) ) ;
#23698=VECTOR ( 'NONE', #37074, 39.37007874015748854 ) ;
#23714=EDGE_CURVE ( 'NONE', #25679, #41157, #26242, .T. ) ;
#23716=ORIENTED_EDGE ( 'NONE', *, *, #26913, .T. ) ;
#23748=CARTESIAN_POINT ( 'NONE',  ( 0.2066929133858268486, 0.7443365962042343131, -3.523993443072799270 ) ) ;
#23767=FILL_AREA_STYLE_COLOUR ( '', #10065 ) ;
#23855=( GEOMETRIC_REPRESENTATION_CONTEXT ( 3 ) GLOBAL_UNCERTAINTY_ASSIGNED_CONTEXT ( ( #46437 ) ) GLOBAL_UNIT_ASSIGNED_CONTEXT ( ( #34333, #1463, #34810 ) ) REPRESENTATION_CONTEXT ( 'NONE', 'WORKASPACE' ) ) ;
#23868=CARTESIAN_POINT ( 'NONE',  ( 0.1527862493557218537, -0.4068158579509408290, -0.9303620633370848214 ) ) ;
#23893=ORIENTED_EDGE ( 'NONE', *, *, #19757, .F. ) ;
#23897=CIRCLE ( 'NONE', #9358, 0.7972440944881888925 ) ;
#23910=DIRECTION ( 'NONE',  ( 0.000000000000000000, 0.000000000000000000, 1.000000000000000000 ) ) ;
#23918=CYLINDRICAL_SURFACE ( 'NONE', #1195, 0.4404574800679669777 ) ;
#23931=DIRECTION ( 'NONE',  ( 0.000000000000000000, 8.979745052115236376E-16, 1.000000000000000000 ) ) ;
#23976=VECTOR ( 'NONE', #4385, 39.37007874015748143 ) ;
#23988=DIRECTION ( 'NONE',  ( 0.000000000000000000, -0.7880107536067207930, 0.6156614753256598460 ) ) ;
#23998=DIRECTION ( 'NONE',  ( 0.000000000000000000, 0.000000000000000000, 1.000000000000000000 ) ) ;
#24015=ORIENTED_EDGE ( 'NONE', *, *, #7160, .F. ) ;
#24067=DIRECTION ( 'NONE',  ( 0.000000000000000000, -0.9699617890481188054, -0.2432573283306645462 ) ) ;
#24114=CARTESIAN_POINT ( 'NONE',  ( 0.1574803149606300023, 0.7443365962042343131, -3.523993443072799270 ) ) ;
#24118=CARTESIAN_POINT ( 'NONE',  ( 0.1476377952755906220, 2.117069812090769609, -1.766975050165344951 ) ) ;
#24134=CARTESIAN_POINT ( 'NONE',  ( 0.1574803149606300023, 0.5323553679591566112, -0.7566348232351033376 ) ) ;
#24137=CARTESIAN_POINT ( 'NONE',  ( -0.2066929133858267931, -0.2714884749021747590, -1.284167712019358198 ) ) ;
#24147=CARTESIAN_POINT ( 'NONE',  ( -0.1476377952755905387, 1.117014023967196179, -3.442880580079819008 ) ) ;
#24192=VERTEX_POINT ( 'NONE', #16107 ) ;
#24241=EDGE_CURVE ( 'NONE', #10554, #47128, #44032, .T. ) ;
#24251=CARTESIAN_POINT ( 'NONE',  ( 0.1574803149606300023, -0.9875035750853327077, -1.463737590216208861 ) ) ;
#24299=DIRECTION ( 'NONE',  ( 0.000000000000000000, -0.9699617890481200266, -0.2432573283306594947 ) ) ;
#24309=ORIENTED_EDGE ( 'NONE', *, *, #18239, .F. ) ;
#24311=CARTESIAN_POINT ( 'NONE',  ( -0.1476377952755905387, 0.5419727308409664213, -0.7545416139885205986 ) ) ;
#24372=ORIENTED_EDGE ( 'NONE', *, *, #41849, .T. ) ;
#24382=DIRECTION ( 'NONE',  ( 1.000000000000000000, 0.000000000000000000, 0.000000000000000000 ) ) ;
#24400=CYLINDRICAL_SURFACE ( 'NONE', #28563, 0.04921259842519680461 ) ;
#24413=AXIS2_PLACEMENT_3D ( 'NONE', #33475, #18359, #25801 ) ;
#24466=ORIENTED_EDGE ( 'NONE', *, *, #33481, .T. ) ;
#24475=EDGE_CURVE ( 'NONE', #5435, #1272, #7930, .T. ) ;
#24480=ORIENTED_EDGE ( 'NONE', *, *, #23714, .T. ) ;
#24507=DIRECTION ( 'NONE',  ( 1.000000000000000000, 0.000000000000000000, 0.000000000000000000 ) ) ;
#24527=DIRECTION ( 'NONE',  ( 1.000000000000000000, -0.000000000000000000, -0.000000000000000000 ) ) ;
#24540=VECTOR ( 'NONE', #37846, 39.37007874015748143 ) ;
#24548=DIRECTION ( 'NONE',  ( 0.000000000000000000, 0.9771240687918540946, 0.2126700594527874133 ) ) ;
#24578=ORIENTED_EDGE ( 'NONE', *, *, #8998, .T. ) ;
#24607=AXIS2_PLACEMENT_3D ( 'NONE', #43758, #11420, #25332 ) ;
#24625=ADVANCED_FACE ( 'NONE', ( #9603 ), #1786, .T. ) ;
#24635=CARTESIAN_POINT ( 'NONE',  ( -0.2066929133858267931, 0.5419727308409657551, -0.7545416139885203766 ) ) ;
#24652=CARTESIAN_POINT ( 'NONE',  ( 0.1574803149606300023, -0.4812165006432428394, -0.8611016091043821596 ) ) ;
#24656=ORIENTED_EDGE ( 'NONE', *, *, #33754, .F. ) ;
#24670=ORIENTED_EDGE ( 'NONE', *, *, #483, .T. ) ;
#24772=ORIENTED_EDGE ( 'NONE', *, *, #24475, .T. ) ;
#24870=AXIS2_PLACEMENT_3D ( 'NONE', #22294, #29778, #17993 ) ;
#24871=LINE ( 'NONE', #13846, #23087 ) ;
#24924=CARTESIAN_POINT ( 'NONE',  ( -0.1476377952755905387, 0.05639690512153997665, -0.1570009270184610506 ) ) ;
#24982=LINE ( 'NONE', #43407, #38410 ) ;
#25067=ORIENTED_EDGE ( 'NONE', *, *, #43327, .T. ) ;
#25075=EDGE_LOOP ( 'NONE', ( #10895, #43105, #11023, #13641 ) ) ;
#25079=LINE ( 'NONE', #36105, #17994 ) ;
#25111=DIRECTION ( 'NONE',  ( -1.000000000000000000, -0.000000000000000000, -0.000000000000000000 ) ) ;
#25154=EDGE_CURVE ( 'NONE', #30513, #23380, #22247, .T. ) ;
#25266=AXIS2_PLACEMENT_3D ( 'NONE', #24147, #19586, #27043 ) ;
#25267=DIRECTION ( 'NONE',  ( 1.000000000000000000, 0.000000000000000000, -0.000000000000000000 ) ) ;
#25332=DIRECTION ( 'NONE',  ( 0.000000000000000000, 0.000000000000000000, 1.000000000000000000 ) ) ;
#25349=CARTESIAN_POINT ( 'NONE',  ( 0.1574803149606299746, 0.7443365962042343131, -3.523993443072799270 ) ) ;
#25369=AXIS2_PLACEMENT_3D ( 'NONE', #25349, #14324, #39462 ) ;
#25398=DIRECTION ( 'NONE',  ( 0.000000000000000000, 3.469446951953614583E-15, 1.000000000000000000 ) ) ;
#25404=B_SPLINE_CURVE_WITH_KNOTS ( 'NONE', 3,
 ( #1096, #5169, #23160, #23868, #26536, #37778 ),
 .UNSPECIFIED., .F., .F.,
 ( 4, 2, 4 ),
 ( -7.834150686268513193E-06, 0.0001896218827938178436, 0.0003870779162739032618 ),
 .UNSPECIFIED. ) ;
#25428=ORIENTED_EDGE ( 'NONE', *, *, #12423, .T. ) ;
#25447=DIRECTION ( 'NONE',  ( -0.000000000000000000, 0.7880107536067207930, -0.6156614753256598460 ) ) ;
#25452=ORIENTED_EDGE ( 'NONE', *, *, #38813, .F. ) ;
#25454=ORIENTED_EDGE ( 'NONE', *, *, #22498, .T. ) ;
#25482=DIRECTION ( 'NONE',  ( 0.000000000000000000, 0.9771240687918540946, 0.2126700594527874133 ) ) ;
#25590=DIRECTION ( 'NONE',  ( 0.000000000000000000, 0.9771240687918510970, 0.2126700594528006527 ) ) ;
#25608=EDGE_LOOP ( 'NONE', ( #41835, #15245, #46916, #67 ) ) ;
#25621=CARTESIAN_POINT ( 'NONE',  ( -0.1673228346456692994, 0.06415291647593684976, -0.1630605872086742514 ) ) ;
#25630=VERTEX_POINT ( 'NONE', #43044 ) ;
#25650=ORIENTED_EDGE ( 'NONE', *, *, #47402, .T. ) ;
#25679=VERTEX_POINT ( 'NONE', #15263 ) ;
#25680=CIRCLE ( 'NONE', #4983, 0.009842519685039376881 ) ;
#25681=AXIS2_PLACEMENT_3D ( 'NONE', #39965, #3074, #29262 ) ;
#25687=AXIS2_PLACEMENT_3D ( 'NONE', #21123, #18248, #29329 ) ;
#25692=CARTESIAN_POINT ( 'NONE',  ( 0.000000000000000000, 0.000000000000000000, 0.000000000000000000 ) ) ;
#25723=FACE_OUTER_BOUND ( 'NONE', #45370, .T. ) ;
#25724=VERTEX_POINT ( 'NONE', #10968 ) ;
#25750=CARTESIAN_POINT ( 'NONE',  ( -0.2066929133858267931, -0.2274162997038020051, -0.9219983537151217323 ) ) ;
#25766=DIRECTION ( 'NONE',  ( 0.000000000000000000, 0.2126700594527834998, -0.9771240687918549828 ) ) ;
#25801=DIRECTION ( 'NONE',  ( 0.000000000000000000, 0.000000000000000000, -1.000000000000000000 ) ) ;
#25820=CYLINDRICAL_SURFACE ( 'NONE', #18700, 0.04921259842519678379 ) ;
#25891=ORIENTED_EDGE ( 'NONE', *, *, #45438, .F. ) ;
#25906=CARTESIAN_POINT ( 'NONE',  ( 0.2018787443954609129, -0.3516577756781031350, -1.037265999283336182 ) ) ;
#25910=VERTEX_POINT ( 'NONE', #22911 ) ;
#25957=VECTOR ( 'NONE', #27289, 39.37007874015748854 ) ;
#26003=CARTESIAN_POINT ( 'NONE',  ( -0.1661139969171220310, -0.4376765877502337143, -0.9700607378021975924 ) ) ;
#26034=ORIENTED_EDGE ( 'NONE', *, *, #22414, .F. ) ;
#26068=CYLINDRICAL_SURFACE ( 'NONE', #41995, 0.04921259842519688787 ) ;
#26080=CARTESIAN_POINT ( 'NONE',  ( 0.2066929133858268486, -0.5175744617845222662, -0.9076376772307633845 ) ) ;
#26109=FACE_OUTER_BOUND ( 'NONE', #16588, .T. ) ;
#26114=CARTESIAN_POINT ( 'NONE',  ( -0.1574803149606299191, 0.06245656531175266396, -0.1492449156640648644 ) ) ;
#26145=DIRECTION ( 'NONE',  ( 0.000000000000000000, 0.6156614753256609562, 0.7880107536067200158 ) ) ;
#26157=CIRCLE ( 'NONE', #37596, 0.04921259842519686706 ) ;
#26174=CARTESIAN_POINT ( 'NONE',  ( -0.2066929133858267931, -0.9875035750853327077, -1.463737590216208861 ) ) ;
#26194=TOROIDAL_SURFACE ( 'NONE', #11664, 0.01968503937007873988, 0.009842519685039369942 ) ;
#26242=LINE ( 'NONE', #8003, #23976 ) ;
#26251=CARTESIAN_POINT ( 'NONE',  ( -0.1884454360679181650, -0.3999716016534896057, -0.9995191014872203406 ) ) ;
#26355=ORIENTED_EDGE ( 'NONE', *, *, #43327, .F. ) ;
#26357=DIRECTION ( 'NONE',  ( -3.469446951953616950E-15, -0.7880107536067223473, 0.6156614753256577366 ) ) ;
#26377=ORIENTED_EDGE ( 'NONE', *, *, #39739, .F. ) ;
#26399=ORIENTED_EDGE ( 'NONE', *, *, #18356, .T. ) ;
#26401=AXIS2_PLACEMENT_3D ( 'NONE', #12800, #32614, #29030 ) ;
#26418=LINE ( 'NONE', #41691, #8378 ) ;
#26496=CIRCLE ( 'NONE', #45562, 0.009842519685039382085 ) ;
#26536=CARTESIAN_POINT ( 'NONE',  ( 0.1502414035307333140, -0.4075443641102559078, -0.9311509272141711424 ) ) ;
#26549=ADVANCED_FACE ( 'NONE', ( #13898 ), #39747, .T. ) ;
#26557=FACE_OUTER_BOUND ( 'NONE', #25075, .T. ) ;
#26566=CARTESIAN_POINT ( 'NONE',  ( -0.1502419002556872329, -0.4075443641102559633, -0.9311509272141712534 ) ) ;
#26577=DIRECTION ( 'NONE',  ( 0.000000000000000000, -0.6156614753256598460, -0.7880107536067206819 ) ) ;
#26578=ORIENTED_EDGE ( 'NONE', *, *, #264, .F. ) ;
#26619=CARTESIAN_POINT ( 'NONE',  ( 0.1574803149606299746, -0.9875035750853327077, -1.463737590216208861 ) ) ;
#26684=AXIS2_PLACEMENT_3D ( 'NONE', #11763, #4071, #11517 ) ;
#26722=LINE ( 'NONE', #41277, #15909 ) ;
#26744=AXIS2_PLACEMENT_3D ( 'NONE', #12093, #11853, #45119 ) ;
#26773=LINE ( 'NONE', #16223, #15413 ) ;
#26776=AXIS2_PLACEMENT_3D ( 'NONE', #46722, #36446, #13908 ) ;
#26836=DIRECTION ( 'NONE',  ( -1.000000000000000000, -0.000000000000000000, 0.000000000000000000 ) ) ;
#26907=VERTEX_POINT ( 'NONE', #4265 ) ;
#26913=EDGE_CURVE ( 'NONE', #2855, #860, #18240, .T. ) ;
#26938=AXIS2_PLACEMENT_3D ( 'NONE', #859, #156, #19078 ) ;
#27019=CARTESIAN_POINT ( 'NONE',  ( 0.1574803149606300023, 0.3648440108500931589, -3.619166627704266670 ) ) ;
#27043=DIRECTION ( 'NONE',  ( 0.000000000000000000, -0.9771240687918510970, -0.2126700594528006527 ) ) ;
#27045=CARTESIAN_POINT ( 'NONE',  ( -0.2066929133858267931, -0.2274162997038020051, -0.9219983537151217323 ) ) ;
#27053=VECTOR ( 'NONE', #19844, 39.37007874015748854 ) ;
#27087=LINE ( 'NONE', #22988, #20304 ) ;
#27135=AXIS2_PLACEMENT_3D ( 'NONE', #12256, #38117, #23269 ) ;
#27140=DIRECTION ( 'NONE',  ( -0.000000000000000000, 0.7880107536067207930, -0.6156614753256597350 ) ) ;
#27159=LINE ( 'NONE', #41712, #45104 ) ;
#27162=DIRECTION ( 'NONE',  ( 0.000000000000000000, 0.6156614753256602901, 0.7880107536067203489 ) ) ;
#27170=EDGE_LOOP ( 'NONE', ( #46482, #38306, #30372, #12288, #9167, #25428 ) ) ;
#27197=AXIS2_PLACEMENT_3D ( 'NONE', #23670, #2314, #23910 ) ;
#27216=LINE ( 'NONE', #41767, #34047 ) ;
#27289=DIRECTION ( 'NONE',  ( 0.000000000000000000, -0.6156614753256597350, -0.7880107536067206819 ) ) ;
#27326=DIRECTION ( 'NONE',  ( 0.000000000000000000, 0.000000000000000000, 1.000000000000000000 ) ) ;
#27362=ORIENTED_EDGE ( 'NONE', *, *, #6330, .F. ) ;
#27452=DIRECTION ( 'NONE',  ( 0.000000000000000000, -0.2432573283306595224, 0.9699617890481201377 ) ) ;
#27471=DIRECTION ( 'NONE',  ( 0.000000000000000000, 0.9771240687918550938, 0.2126700594527823895 ) ) ;
#27478=DIRECTION ( 'NONE',  ( 0.000000000000000000, 0.2126700594527800581, -0.9771240687918557599 ) ) ;
#27481=CIRCLE ( 'NONE', #39661, 0.009842519685039354330 ) ;
#27527=CARTESIAN_POINT ( 'NONE',  ( -0.1968503937007874127, 0.09275486626281861935, -0.1104648588920805335 ) ) ;
#27628=PLANE ( 'NONE',  #47401 ) ;
#27637=EDGE_CURVE ( 'NONE', #25679, #42397, #40442, .T. ) ;
#27771=VECTOR ( 'NONE', #33267, 39.37007874015748143 ) ;
#27805=EDGE_CURVE ( 'NONE', #28092, #8495, #25404, .T. ) ;
#27847=EDGE_CURVE ( 'NONE', #17869, #46334, #16685, .T. ) ;
#27932=DIRECTION ( 'NONE',  ( -0.000000000000000000, 0.6156614753256597350, 0.7880107536067206819 ) ) ;
#27976=EDGE_LOOP ( 'NONE', ( #9375, #44605, #43116, #45625 ) ) ;
#27981=TOROIDAL_SURFACE ( 'NONE', #11896, 0.7972440944881888925, 0.009842519685039369942 ) ;
#28001=CARTESIAN_POINT ( 'NONE',  ( -0.1574803149606299191, -0.9875035750853327077, -1.463737590216208861 ) ) ;
#28011=EDGE_LOOP ( 'NONE', ( #30218, #18794, #13975, #20011 ) ) ;
#28015=DIRECTION ( 'NONE',  ( -1.000000000000000000, -0.000000000000000000, 0.000000000000000000 ) ) ;
#28027=ORIENTED_EDGE ( 'NONE', *, *, #28209, .T. ) ;
#28054=CYLINDRICAL_SURFACE ( 'NONE', #18063, 0.009842519685039376881 ) ;
#28069=ADVANCED_FACE ( 'NONE', ( #35370 ), #46596, .T. ) ;
#28092=VERTEX_POINT ( 'NONE', #39399 ) ;
#28151=ORIENTED_EDGE ( 'NONE', *, *, #8699, .F. ) ;
#28153=ORIENTED_EDGE ( 'NONE', *, *, #7315, .T. ) ;
#28163=EDGE_CURVE ( 'NONE', #7550, #8597, #4163, .T. ) ;
#28167=CARTESIAN_POINT ( 'NONE',  ( 0.1574803149606299746, 0.7443365962042343131, -3.523993443072799270 ) ) ;
#28190=VERTEX_POINT ( 'NONE', #33439 ) ;
#28209=EDGE_CURVE ( 'NONE', #15230, #17877, #27481, .T. ) ;
#28221=VERTEX_POINT ( 'NONE', #87 ) ;
#28255=AXIS2_PLACEMENT_3D ( 'NONE', #1363, #34699, #1127 ) ;
#28277=FACE_OUTER_BOUND ( 'NONE', #4624, .T. ) ;
#28305=VERTEX_POINT ( 'NONE', #3703 ) ;
#28316=CARTESIAN_POINT ( 'NONE',  ( -0.1574803149606299191, -0.2237541348899642346, -1.272196386806234925 ) ) ;
#28393=CIRCLE ( 'NONE', #36789, 0.009842519685039378616 ) ;
#28416=EDGE_CURVE ( 'NONE', #25910, #33099, #46616, .T. ) ;
#28457=ORIENTED_EDGE ( 'NONE', *, *, #38527, .F. ) ;
#28481=FACE_OUTER_BOUND ( 'NONE', #22214, .T. ) ;
#28486=VECTOR ( 'NONE', #7643, 39.37007874015748854 ) ;
#28495=PLANE ( 'NONE',  #19194 ) ;
#28498=ADVANCED_FACE ( 'NONE', ( #23104 ), #36681, .T. ) ;
#28563=AXIS2_PLACEMENT_3D ( 'NONE', #16972, #2341, #31379 ) ;
#28574=AXIS2_PLACEMENT_3D ( 'NONE', #26174, #16042, #11318 ) ;
#28582=ORIENTED_EDGE ( 'NONE', *, *, #21973, .F. ) ;
#28639=ORIENTED_EDGE ( 'NONE', *, *, #16994, .F. ) ;
#28689=EDGE_LOOP ( 'NONE', ( #26399, #4546, #40524, #45490 ) ) ;
#28708=VERTEX_POINT ( 'NONE', #16624 ) ;
#28709=DIRECTION ( 'NONE',  ( -0.000000000000000000, -0.2432573283306646017, 0.9699617890481188054 ) ) ;
#28764=CARTESIAN_POINT ( 'NONE',  ( 0.1574803149606299746, -0.4410959923581754816, -0.9673892061308019263 ) ) ;
#28782=ORIENTED_EDGE ( 'NONE', *, *, #27805, .T. ) ;
#28890=ORIENTED_EDGE ( 'NONE', *, *, #21603, .T. ) ;
#28894=DIRECTION ( 'NONE',  ( -1.000000000000000000, -0.000000000000000000, 0.000000000000000000 ) ) ;
#28912=CARTESIAN_POINT ( 'NONE',  ( -0.1476377952755905387, 0.7443365962042343131, -3.523993443072799270 ) ) ;
#29030=DIRECTION ( 'NONE',  ( 0.000000000000000000, 0.000000000000000000, 1.000000000000000000 ) ) ;
#29069=CIRCLE ( 'NONE', #29852, 0.009842519685039361269 ) ;
#29171=DIRECTION ( 'NONE',  ( -0.000000000000000000, 0.6156614753256608452, 0.7880107536067200158 ) ) ;
#29207=EDGE_CURVE ( 'NONE', #12477, #41019, #26418, .T. ) ;
#29221=EDGE_CURVE ( 'NONE', #12477, #25910, #35179, .T. ) ;
#29226=DIRECTION ( 'NONE',  ( 0.000000000000000000, -0.7880107536067200158, 0.6156614753256608452 ) ) ;
#29228=CARTESIAN_POINT ( 'NONE',  ( -0.2066929133858267931, 1.174718201258053485, -3.430321324600322352 ) ) ;
#29262=DIRECTION ( 'NONE',  ( 0.000000000000000000, 0.6156614753256595129, 0.7880107536067211260 ) ) ;
#29298=ORIENTED_EDGE ( 'NONE', *, *, #19719, .F. ) ;
#29301=VERTEX_POINT ( 'NONE', #46483 ) ;
#29316=CARTESIAN_POINT ( 'NONE',  ( 0.1661702112335584902, -0.4376325038317900873, -0.9700951799340379322 ) ) ;
#29329=DIRECTION ( 'NONE',  ( 0.000000000000000000, 0.7880107536067206819, -0.6156614753256598460 ) ) ;
#29351=ORIENTED_EDGE ( 'NONE', *, *, #6330, .T. ) ;
#29373=PRODUCT_DEFINITION_CONTEXT ( 'detailed design', #13765, 'design' ) ;
#29405=DIRECTION ( 'NONE',  ( -1.000000000000000000, -0.000000000000000000, -0.000000000000000000 ) ) ;
#29419=VECTOR ( 'NONE', #18888, 39.37007874015748854 ) ;
#29436=ORIENTED_EDGE ( 'NONE', *, *, #8423, .T. ) ;
#29447=EDGE_CURVE ( 'NONE', #2867, #43605, #17543, .T. ) ;
#29450=CARTESIAN_POINT ( 'NONE',  ( -0.1574803149606299191, 0.09445121742700228473, -0.1242805304366905728 ) ) ;
#29477=LINE ( 'NONE', #36845, #23698 ) ;
#29494=DIRECTION ( 'NONE',  ( 1.000000000000000000, 0.000000000000000000, 0.000000000000000000 ) ) ;
#29496=EDGE_CURVE ( 'NONE', #15230, #20344, #22044, .T. ) ;
#29512=TOROIDAL_SURFACE ( 'NONE', #33316, 0.03937007874015747977, 0.009842519685039369942 ) ;
#29533=ORIENTED_EDGE ( 'NONE', *, *, #847, .F. ) ;
#29574=DIRECTION ( 'NONE',  ( 0.000000000000000000, -0.6156614753256597350, -0.7880107536067207930 ) ) ;
#29620=EDGE_LOOP ( 'NONE', ( #6725, #10707, #35852, #22298 ) ) ;
#29653=ADVANCED_FACE ( 'NONE', ( #32130 ), #46967, .F. ) ;
#29689=LINE ( 'NONE', #40859, #41403 ) ;
#29729=EDGE_CURVE ( 'NONE', #25910, #18185, #4278, .T. ) ;
#29769=DIRECTION ( 'NONE',  ( 0.000000000000000000, -0.6156614753256619554, -0.7880107536067190166 ) ) ;
#29778=DIRECTION ( 'NONE',  ( 0.000000000000000000, -0.9699617890481188054, -0.2432573283306646017 ) ) ;
#29844=VECTOR ( 'NONE', #47455, 39.37007874015748854 ) ;
#29852=AXIS2_PLACEMENT_3D ( 'NONE', #37929, #30524, #44378 ) ;
#29866=DIRECTION ( 'NONE',  ( 0.000000000000000000, 0.2432573283306645739, -0.9699617890481188054 ) ) ;
#29954=EDGE_LOOP ( 'NONE', ( #1877, #4539, #22299, #24372 ) ) ;
#29959=ORIENTED_EDGE ( 'NONE', *, *, #16824, .F. ) ;
#29974=DIRECTION ( 'NONE',  ( -0.000000000000000000, -0.6156614753256586248, -0.7880107536067217922 ) ) ;
#30010=CARTESIAN_POINT ( 'NONE',  ( 0.1595021679387737257, -0.4410959923581755371, -0.9673892061308022594 ) ) ;
#30020=CIRCLE ( 'NONE', #23072, 0.009842519685039382085 ) ;
#30092=VERTEX_POINT ( 'NONE', #24652 ) ;
#30134=ORIENTED_EDGE ( 'NONE', *, *, #14679, .F. ) ;
#30151=PRODUCT_DEFINITION_FORMATION_WITH_SPECIFIED_SOURCE ( 'ANY', '', #46114, .NOT_KNOWN. ) ;
#30153=DIRECTION ( 'NONE',  ( 0.000000000000000000, 0.7880107536067233465, -0.6156614753256566264 ) ) ;
#30170=LINE ( 'NONE', #37300, #8405 ) ;
#30173=DIRECTION ( 'NONE',  ( 0.000000000000000000, -0.7880107536067206819, 0.6156614753256597350 ) ) ;
#30184=CARTESIAN_POINT ( 'NONE',  ( 0.1574803149606300023, 0.07021257666614932891, -0.1553045758542778432 ) ) ;
#30185=CARTESIAN_POINT ( 'NONE',  ( -0.1527872282172904050, -0.4068155598699056963, -0.9303617405735025159 ) ) ;
#30190=DIRECTION ( 'NONE',  ( 5.403967543462346582E-15, -0.6156614753256592909, -0.7880107536067211260 ) ) ;
#30216=LINE ( 'NONE', #22032, #44549 ) ;
#30218=ORIENTED_EDGE ( 'NONE', *, *, #39739, .T. ) ;
#30220=CARTESIAN_POINT ( 'NONE',  ( 0.1574803149606299746, -0.2274162997038020051, -0.9219983537151217323 ) ) ;
#30242=LINE ( 'NONE', #37624, #45514 ) ;
#30244=CARTESIAN_POINT ( 'NONE',  ( 0.1574803149606300023, 0.1005108776172155827, -0.1165245190822938037 ) ) ;
#30254=ORIENTED_EDGE ( 'NONE', *, *, #38107, .F. ) ;
#30319=EDGE_CURVE ( 'NONE', #43605, #2855, #30170, .T. ) ;
#30325=CYLINDRICAL_SURFACE ( 'NONE', #9316, 0.009842519685039428923 ) ;
#30331=VERTEX_POINT ( 'NONE', #18620 ) ;
#30338=CARTESIAN_POINT ( 'NONE',  ( 0.2066929133858268486, 0.5419727308409655331, -0.7545416139885203766 ) ) ;
#30354=EDGE_CURVE ( 'NONE', #6659, #30331, #4555, .T. ) ;
#30372=ORIENTED_EDGE ( 'NONE', *, *, #32823, .T. ) ;
#30388=DIRECTION ( 'NONE',  ( -0.000000000000000000, -0.2432573283306646017, 0.9699617890481188054 ) ) ;
#30390=DIRECTION ( 'NONE',  ( -0.000000000000000000, 0.7880107536067207930, -0.6156614753256597350 ) ) ;
#30412=CYLINDRICAL_SURFACE ( 'NONE', #25266, 0.009842519685039428923 ) ;
#30415=DIRECTION ( 'NONE',  ( 0.000000000000000000, -0.7880107536067207930, 0.6156614753256598460 ) ) ;
#30495=DIRECTION ( 'NONE',  ( -0.000000000000000000, 0.7880107536067207930, -0.6156614753256598460 ) ) ;
#30509=DIRECTION ( 'NONE',  ( 0.000000000000000000, -0.6156614753256597350, -0.7880107536067207930 ) ) ;
#30513=VERTEX_POINT ( 'NONE', #24134 ) ;
#30524=DIRECTION ( 'NONE',  ( 1.000000000000000000, 0.000000000000000000, -0.000000000000000000 ) ) ;
#30552=VECTOR ( 'NONE', #44120, 39.37007874015748854 ) ;
#30566=PLANE ( 'NONE',  #13075 ) ;
#30627=CARTESIAN_POINT ( 'NONE',  ( 0.2066929133858268486, 0.3648440108500932699, -3.619166627704267114 ) ) ;
#30639=CARTESIAN_POINT ( 'NONE',  ( -0.1476377952755905387, -0.4075443641102559078, -0.9311509272141712534 ) ) ;
#30649=ORIENTED_EDGE ( 'NONE', *, *, #4967, .F. ) ;
#30666=ORIENTED_EDGE ( 'NONE', *, *, #37045, .F. ) ;
#30668=EDGE_CURVE ( 'NONE', #30331, #2867, #35152, .T. ) ;
#30688=CARTESIAN_POINT ( 'NONE',  ( 0.2066929133858268486, -0.5175744617845221551, -0.9076376772307632734 ) ) ;
#30747=SURFACE_STYLE_USAGE ( .BOTH. , #23542 ) ;
#30869=DIRECTION ( 'NONE',  ( 0.000000000000000000, 0.2432573283306646017, -0.9699617890481188054 ) ) ;
#30891=ORIENTED_EDGE ( 'NONE', *, *, #18701, .F. ) ;
#30904=FACE_BOUND ( 'NONE', #46606, .T. ) ;
#30907=PLANE ( 'NONE',  #41499 ) ;
#30948=EDGE_LOOP ( 'NONE', ( #28027, #22111, #2778, #35840 ) ) ;
#30967=ORIENTED_EDGE ( 'NONE', *, *, #17917, .T. ) ;
#30974=DIRECTION ( 'NONE',  ( -1.000000000000000000, -0.000000000000000000, -0.000000000000000000 ) ) ;
#31055=CIRCLE ( 'NONE', #43252, 0.4404574800679669777 ) ;
#31063=ORIENTED_EDGE ( 'NONE', *, *, #23714, .F. ) ;
#31076=CIRCLE ( 'NONE', #13442, 0.4404574800679669777 ) ;
#31093=CIRCLE ( 'NONE', #32525, 0.4404574800679669777 ) ;
#31117=AXIS2_PLACEMENT_3D ( 'NONE', #5046, #19426, #44338 ) ;
#31125=DIRECTION ( 'NONE',  ( 0.000000000000000000, 0.000000000000000000, 1.000000000000000000 ) ) ;
#31181=CARTESIAN_POINT ( 'NONE',  ( 0.1574803149606299746, -0.2274162997038020051, -0.9219983537151217323 ) ) ;
#31272=CARTESIAN_POINT ( 'NONE',  ( 0.2066929133858268486, 0.7443365962042343131, -3.523993443072799270 ) ) ;
#31286=CARTESIAN_POINT ( 'NONE',  ( 0.1574803149606299746, 0.5419727308409655331, -0.7545416139885203766 ) ) ;
#31334=AXIS2_PLACEMENT_3D ( 'NONE', #31286, #12840, #27471 ) ;
#31379=DIRECTION ( 'NONE',  ( 0.000000000000000000, 0.6156614753256578476, 0.7880107536067223473 ) ) ;
#31414=EDGE_CURVE ( 'NONE', #41019, #45599, #5830, .T. ) ;
#31422=CARTESIAN_POINT ( 'NONE',  ( 0.1476377952755906220, -0.4812165006432430059, -0.8611016091043821596 ) ) ;
#31455=CIRCLE ( 'NONE', #39080, 0.7775590551181102983 ) ;
#31510=AXIS2_PLACEMENT_3D ( 'NONE', #42575, #1626, #38299 ) ;
#31575=VECTOR ( 'NONE', #42685, 39.37007874015748854 ) ;
#31583=DIRECTION ( 'NONE',  ( 0.000000000000000000, 0.000000000000000000, -1.000000000000000000 ) ) ;
#31593=CARTESIAN_POINT ( 'NONE',  ( -0.1574803149606299191, 0.1005108776172155410, -0.1165245190822937899 ) ) ;
#31612=PRODUCT_DEFINITION_SHAPE ( 'NONE', 'NONE',  #7809 ) ;
#31778=CARTESIAN_POINT ( 'NONE',  ( 0.1574803149606299746, 0.3171096708378827178, -3.631137952917390166 ) ) ;
#31779=EDGE_CURVE ( 'NONE', #6124, #7028, #42898, .T. ) ;
#31881=ORIENTED_EDGE ( 'NONE', *, *, #32823, .F. ) ;
#31928=DIRECTION ( 'NONE',  ( 1.000000000000000000, 0.000000000000000000, -0.000000000000000000 ) ) ;
#31942=EDGE_CURVE ( 'NONE', #29301, #28190, #5173, .T. ) ;
#31954=CARTESIAN_POINT ( 'NONE',  ( -0.1476377952755905387, -0.4933358210236689634, -0.8766136318131756422 ) ) ;
#31973=DIRECTION ( 'NONE',  ( -1.000000000000000000, -0.000000000000000000, 0.000000000000000000 ) ) ;
#32009=DIRECTION ( 'NONE',  ( 0.000000000000000000, 0.7880107536067200158, -0.6156614753256608452 ) ) ;
#32024=EDGE_CURVE ( 'NONE', #28708, #24192, #26773, .T. ) ;
#32050=ADVANCED_FACE ( 'NONE', ( #41333 ), #22033, .T. ) ;
#32073=ORIENTED_EDGE ( 'NONE', *, *, #18705, .T. ) ;
#32077=CARTESIAN_POINT ( 'NONE',  ( -0.1476377952755905387, -0.4812165006432425063, -0.8611016091043822707 ) ) ;
#32097=EDGE_CURVE ( 'NONE', #42397, #30513, #31455, .T. ) ;
#32130=FACE_OUTER_BOUND ( 'NONE', #10177, .T. ) ;
#32145=DIRECTION ( 'NONE',  ( 0.000000000000000000, -0.9699617890481186944, -0.2432573283306648515 ) ) ;
#32179=TOROIDAL_SURFACE ( 'NONE', #42093, 0.03937007874015747977, 0.009842519685039369942 ) ;
#32218=ADVANCED_FACE ( 'NONE', ( #45649 ), #17372, .F. ) ;
#32253=CIRCLE ( 'NONE', #8494, 0.01968503937007874335 ) ;
#32296=CIRCLE ( 'NONE', #24607, 0.3912448816427701037 ) ;
#32355=VECTOR ( 'NONE', #19279, 39.37007874015748143 ) ;
#32480=ADVANCED_BREP_SHAPE_REPRESENTATION ( 'Link Bar', ( #21111, #20860 ), #6323 ) ;
#32484=ADVANCED_FACE ( 'NONE', ( #12450, #30904 ), #34956, .T. ) ;
#32525=AXIS2_PLACEMENT_3D ( 'NONE', #28167, #28894, #47058 ) ;
#32541=FACE_OUTER_BOUND ( 'NONE', #33836, .T. ) ;
#32588=CARTESIAN_POINT ( 'NONE',  ( 0.1476377952755906220, 0.07627223685636320971, -0.1475485644998805468 ) ) ;
#32589=DIRECTION ( 'NONE',  ( 0.000000000000000000, 0.000000000000000000, -1.000000000000000000 ) ) ;
#32614=DIRECTION ( 'NONE',  ( -1.000000000000000000, -0.000000000000000000, 0.000000000000000000 ) ) ;
#32619=VECTOR ( 'NONE', #25111, 39.37007874015748143 ) ;
#32644=FACE_OUTER_BOUND ( 'NONE', #41155, .T. ) ;
#32652=DIRECTION ( 'NONE',  ( 0.000000000000000000, 0.000000000000000000, 1.000000000000000000 ) ) ;
#32716=ADVANCED_FACE ( 'NONE', ( #14081 ), #11608, .T. ) ;
#32823=EDGE_CURVE ( 'NONE', #35433, #2521, #37712, .T. ) ;
#32824=ADVANCED_FACE ( 'NONE', ( #5338 ), #30325, .F. ) ;
#32841=B_SPLINE_CURVE_WITH_KNOTS ( 'NONE', 3,
 ( #568, #4885, #41282, #11390, #346, #22639, #26251, #22391, #44188, #7775, #8482, #26003, #1285, #4396, #37244, #8010 ),
 .UNSPECIFIED., .F., .F.,
 ( 4, 2, 2, 2, 2, 2, 2, 4 ),
 ( 0.000000000000000000, 0.001193518611021448031, 0.002387037222042896062, 0.003580555833064344093, 0.004177315138575062904, 0.004475694791330420141, 0.004624884617708099194, 0.004774074444085778246 ),
 .UNSPECIFIED. ) ;
#32846=VECTOR ( 'NONE', #5196, 39.37007874015748854 ) ;
#32864=ORIENTED_EDGE ( 'NONE', *, *, #32024, .F. ) ;
#32876=ORIENTED_EDGE ( 'NONE', *, *, #22835, .T. ) ;
#32886=VECTOR ( 'NONE', #618, 39.37007874015748143 ) ;
#32942=LINE ( 'NONE', #43203, #19057 ) ;
#32977=DIRECTION ( 'NONE',  ( 0.000000000000000000, -0.7880107536067200158, 0.6156614753256608452 ) ) ;
#32986=CIRCLE ( 'NONE', #42135, 0.04921259842519683236 ) ;
#33036=DIRECTION ( 'NONE',  ( -0.000000000000000000, 0.7880107536067207930, -0.6156614753256598460 ) ) ;
#33047=STYLED_ITEM ( 'NONE', ( #18576 ), #21111 ) ;
#33057=DIRECTION ( 'NONE',  ( 1.944138416145897342E-15, -0.6156614753256602901, -0.7880107536067203489 ) ) ;
#33085=DIRECTION ( 'NONE',  ( 0.000000000000000000, 0.2432573283306646017, -0.9699617890481188054 ) ) ;
#33099=VERTEX_POINT ( 'NONE', #13718 ) ;
#33125=CIRCLE ( 'NONE', #7833, 0.009842519685039428923 ) ;
#33201=DIRECTION ( 'NONE',  ( -0.000000000000000000, 0.7880107536067207930, -0.6156614753256598460 ) ) ;
#33243=FACE_OUTER_BOUND ( 'NONE', #13578, .T. ) ;
#33267=DIRECTION ( 'NONE',  ( 1.000000000000000000, 0.000000000000000000, 0.000000000000000000 ) ) ;
#33280=DIRECTION ( 'NONE',  ( -3.375873585268818961E-16, -0.2432573283306649070, 0.9699617890481186944 ) ) ;
#33305=EDGE_CURVE ( 'NONE', #34485, #43921, #24982, .T. ) ;
#33316=AXIS2_PLACEMENT_3D ( 'NONE', #11958, #12434, #26577 ) ;
#33351=AXIS2_PLACEMENT_3D ( 'NONE', #42333, #16712, #31583 ) ;
#33355=CARTESIAN_POINT ( 'NONE',  ( 0.2056049205965837234, -0.3271121446598783677, -1.056443147991412923 ) ) ;
#33361=ORIENTED_EDGE ( 'NONE', *, *, #30319, .F. ) ;
#33413=CIRCLE ( 'NONE', #31117, 0.7874015748031495399 ) ;
#33439=CARTESIAN_POINT ( 'NONE',  ( -0.2066929133858267931, 0.2573565155132529481, -0.3015174453633730489 ) ) ;
#33450=EDGE_LOOP ( 'NONE', ( #2030, #46775, #29298, #12077 ) ) ;
#33475=CARTESIAN_POINT ( 'NONE',  ( -0.2066929133858267931, -0.5115148015943089543, -0.8998816658763667542 ) ) ;
#33481=EDGE_CURVE ( 'NONE', #41157, #6624, #5286, .T. ) ;
#33504=ORIENTED_EDGE ( 'NONE', *, *, #42120, .F. ) ;
#33508=LINE ( 'NONE', #34219, #9649 ) ;
#33541=CARTESIAN_POINT ( 'NONE',  ( -0.2066929133858267931, -0.9875035750853327077, -1.463737590216208861 ) ) ;
#33553=CARTESIAN_POINT ( 'NONE',  ( 0.2066929133858268486, -0.2274162997038020051, -0.9219983537151217323 ) ) ;
#33561=CARTESIAN_POINT ( 'NONE',  ( -0.1476377952755905387, -0.4950321721878530035, -0.8627979602685655891 ) ) ;
#33571=EDGE_LOOP ( 'NONE', ( #308, #8736, #25454, #40881, #40595, #5753, #28890, #37664 ) ) ;
#33608=DIRECTION ( 'NONE',  ( -1.000000000000000000, 0.000000000000000000, 0.000000000000000000 ) ) ;
#33628=EDGE_CURVE ( 'NONE', #8992, #30331, #14685, .T. ) ;
#33638=ORIENTED_EDGE ( 'NONE', *, *, #38107, .T. ) ;
#33681=ADVANCED_FACE ( 'NONE', ( #9561 ), #7796, .T. ) ;
#33691=DIRECTION ( 'NONE',  ( -0.000000000000000000, 0.6156614753256598460, 0.7880107536067207930 ) ) ;
#33754=EDGE_CURVE ( 'NONE', #43921, #8495, #24871, .T. ) ;
#33836=EDGE_LOOP ( 'NONE', ( #28153, #30134, #39429, #38249 ) ) ;
#33906=ADVANCED_FACE ( 'NONE', ( #4444 ), #4938, .T. ) ;
#33911=CARTESIAN_POINT ( 'NONE',  ( -0.2066929133858267931, -0.5253304731389190074, -0.9015780170405504057 ) ) ;
#33960=CIRCLE ( 'NONE', #22461, 0.7874015748031495399 ) ;
#33996=FACE_OUTER_BOUND ( 'NONE', #15417, .T. ) ;
#34001=DIRECTION ( 'NONE',  ( 0.000000000000000000, -0.2126700594527834998, 0.9771240687918549828 ) ) ;
#34007=EDGE_CURVE ( 'NONE', #44611, #9478, #36874, .T. ) ;
#34012=EDGE_CURVE ( 'NONE', #35433, #29301, #11264, .T. ) ;
#34032=DIRECTION ( 'NONE',  ( 0.000000000000000000, 0.6156614753256591799, 0.7880107536067213481 ) ) ;
#34047=VECTOR ( 'NONE', #23588, 39.37007874015748854 ) ;
#34091=DIRECTION ( 'NONE',  ( 0.000000000000000000, -0.2126700594527977661, 0.9771240687918517631 ) ) ;
#34168=B_SPLINE_CURVE_WITH_KNOTS ( 'NONE', 3,
 ( #14887, #30010, #11758, #22531, #29316, #7917, #37149, #11294, #18929, #11527, #702, #37377, #25906, #33355, #11064, #15360 ),
 .UNSPECIFIED., .F., .F.,
 ( 4, 2, 2, 2, 2, 2, 2, 4 ),
 ( 0.000000000000000000, 0.0001515175770179333456, 0.0003030351540358666913, 0.0006060703080717382615, 0.001212140616143477607, 0.002424281232286962587, 0.003636421848430447783, 0.004848562464573932980 ),
 .UNSPECIFIED. ) ;
#34172=EDGE_CURVE ( 'NONE', #7028, #26907, #30216, .T. ) ;
#34219=CARTESIAN_POINT ( 'NONE',  ( 0.2066929133858268486, -0.4410959923581754816, -0.9673892061308019263 ) ) ;
#34239=ORIENTED_EDGE ( 'NONE', *, *, #28209, .F. ) ;
#34261=CARTESIAN_POINT ( 'NONE',  ( -0.2066929133858267931, -0.4410959923581754816, -0.9673892061308019263 ) ) ;
#34320=DIRECTION ( 'NONE',  ( 0.000000000000000000, -0.9771240687918510970, -0.2126700594528006527 ) ) ;
#34324=CARTESIAN_POINT ( 'NONE',  ( 0.1476377952755906220, 0.3743908788525358022, -3.616772362661642592 ) ) ;
#34333=( CONVERSION_BASED_UNIT ( 'INCH', #19040 ) LENGTH_UNIT ( ) NAMED_UNIT ( #13025 ) ) ;
#34343=AXIS2_PLACEMENT_3D ( 'NONE', #20111, #46211, #34759 ) ;
#34370=AXIS2_PLACEMENT_3D ( 'NONE', #27045, #8320, #16481 ) ;
#34379=PLANE ( 'NONE',  #2324 ) ;
#34410=AXIS2_PLACEMENT_3D ( 'NONE', #41114, #44479, #22215 ) ;
#34438=TOROIDAL_SURFACE ( 'NONE', #13762, 0.3814023619577306956, 0.009842519685039369942 ) ;
#34485=VERTEX_POINT ( 'NONE', #20792 ) ;
#34488=VERTEX_POINT ( 'NONE', #24635 ) ;
#34532=CIRCLE ( 'NONE', #10811, 0.8366141732283465249 ) ;
#34557=( LENGTH_UNIT ( ) NAMED_UNIT ( * ) SI_UNIT ( $, .METRE. ) ) ;
#34572=CARTESIAN_POINT ( 'NONE',  ( -0.1968503937007874127, 0.06245656531175255294, -0.1492449156640650032 ) ) ;
#34629=ORIENTED_EDGE ( 'NONE', *, *, #483, .F. ) ;
#34644=ORIENTED_EDGE ( 'NONE', *, *, #38052, .T. ) ;
#34667=AXIS2_PLACEMENT_3D ( 'NONE', #15805, #1623, #16272 ) ;
#34699=DIRECTION ( 'NONE',  ( -0.000000000000000000, 0.9771240687918548717, 0.2126700594527834720 ) ) ;
#34709=EDGE_CURVE ( 'NONE', #1718, #2020, #8018, .T. ) ;
#34759=DIRECTION ( 'NONE',  ( 0.000000000000000000, -0.9699617890481172511, -0.2432573283306705969 ) ) ;
#34810=( NAMED_UNIT ( * ) SI_UNIT ( $, .STERADIAN. ) SOLID_ANGLE_UNIT ( ) ) ;
#34820=ORIENTED_EDGE ( 'NONE', *, *, #39731, .T. ) ;
#34869=CARTESIAN_POINT ( 'NONE',  ( -0.1574803149606299191, 0.5419727308409664213, -0.7545416139885205986 ) ) ;
#34916=TOROIDAL_SURFACE ( 'NONE', #10421, 0.7775590551181102983, 0.009842519685039369942 ) ;
#34924=EDGE_CURVE ( 'NONE', #12211, #14871, #11873, .T. ) ;
#34956=PLANE ( 'NONE',  #43701 ) ;
#34973=ORIENTED_EDGE ( 'NONE', *, *, #29729, .T. ) ;
#35000=LINE ( 'NONE', #5747, #42462 ) ;
#35076=ORIENTED_EDGE ( 'NONE', *, *, #5387, .T. ) ;
#35088=DIRECTION ( 'NONE',  ( 0.000000000000000000, 0.2432573283306645462, -0.9699617890481188054 ) ) ;
#35138=DIRECTION ( 'NONE',  ( -1.000000000000000000, -0.000000000000000000, -0.000000000000000000 ) ) ;
#35152=LINE ( 'NONE', #30627, #21410 ) ;
#35177=CARTESIAN_POINT ( 'NONE',  ( -0.2066929133858267931, -0.5221178280460080368, -0.9040880104747088808 ) ) ;
#35179=CIRCLE ( 'NONE', #44318, 0.04921259842519686012 ) ;
#35205=VECTOR ( 'NONE', #37797, 39.37007874015748143 ) ;
#35246=DIRECTION ( 'NONE',  ( -0.000000000000000000, 0.7880107536067207930, -0.6156614753256598460 ) ) ;
#35252=ADVANCED_FACE ( 'NONE', ( #11572 ), #46882, .T. ) ;
#35273=CARTESIAN_POINT ( 'NONE',  ( 0.1574803149606300023, -0.4075443641102559078, -0.9311509272141712534 ) ) ;
#35297=EDGE_CURVE ( 'NONE', #34488, #28708, #43039, .T. ) ;
#35331=AXIS2_PLACEMENT_3D ( 'NONE', #4073, #15123, #29769 ) ;
#35333=CARTESIAN_POINT ( 'NONE',  ( 0.1574803149606299746, 1.174718201258053485, -3.430321324600322352 ) ) ;
#35348=ORIENTED_EDGE ( 'NONE', *, *, #34709, .F. ) ;
#35351=CARTESIAN_POINT ( 'NONE',  ( -0.1574803149606299191, 1.126631386849004990, -3.440787370833234604 ) ) ;
#35353=EDGE_CURVE ( 'NONE', #41157, #39149, #19322, .T. ) ;
#35368=CARTESIAN_POINT ( 'NONE',  ( -0.1574803149606299191, 0.3743908788525360798, -3.616772362661643925 ) ) ;
#35369=DIRECTION ( 'NONE',  ( 0.000000000000000000, 0.000000000000000000, 1.000000000000000000 ) ) ;
#35370=FACE_OUTER_BOUND ( 'NONE', #20399, .T. ) ;
#35416=DIRECTION ( 'NONE',  ( 0.000000000000000000, -1.756682000989171636E-15, 1.000000000000000000 ) ) ;
#35433=VERTEX_POINT ( 'NONE', #12533 ) ;
#35529=( BOUNDED_CURVE ( )  B_SPLINE_CURVE ( 3, ( #26080, #4236, #3564, #8087 ),
 .UNSPECIFIED., .F., .F. ) 
 B_SPLINE_CURVE_WITH_KNOTS ( ( 4, 4 ),
 ( 3.141592653589813544, 4.712388980384689674 ),
 .UNSPECIFIED. ) 
 CURVE ( )  GEOMETRIC_REPRESENTATION_ITEM ( )  RATIONAL_B_SPLINE_CURVE ( ( 1.000000000000000000, 0.8047378541243698225, 0.8047378541243698225, 1.000000000000000000 ) ) 
 REPRESENTATION_ITEM ( '' )  ) ;
#35546=CARTESIAN_POINT ( 'NONE',  ( 0.1476377952755906220, 1.126631386849005878, -3.440787370833236380 ) ) ;
#35601=DIRECTION ( 'NONE',  ( 0.000000000000000000, 0.2432573283306646017, -0.9699617890481188054 ) ) ;
#35622=CIRCLE ( 'NONE', #25681, 0.04921259842519683930 ) ;
#35635=ADVANCED_FACE ( 'NONE', ( #8824 ), #12484, .F. ) ;
#35660=EDGE_CURVE ( 'NONE', #34488, #28305, #22973, .T. ) ;
#35723=DIRECTION ( 'NONE',  ( 1.000000000000000000, 0.000000000000000000, -0.000000000000000000 ) ) ;
#35752=ORIENTED_EDGE ( 'NONE', *, *, #3086, .F. ) ;
#35783=DIRECTION ( 'NONE',  ( 0.000000000000000000, 0.7880107536067200158, -0.6156614753256608452 ) ) ;
#35840=ORIENTED_EDGE ( 'NONE', *, *, #29496, .F. ) ;
#35852=ORIENTED_EDGE ( 'NONE', *, *, #5387, .F. ) ;
#35967=CIRCLE ( 'NONE', #15308, 0.04921259842519691563 ) ;
#36005=DIRECTION ( 'NONE',  ( 0.000000000000000000, 6.938893903907222856E-15, 1.000000000000000000 ) ) ;
#36013=CARTESIAN_POINT ( 'NONE',  ( 0.1574803149606300023, 2.117069812090769609, -1.766975050165344951 ) ) ;
#36040=DIRECTION ( 'NONE',  ( 1.000000000000000000, 0.000000000000000000, 0.000000000000000000 ) ) ;
#36089=ORIENTED_EDGE ( 'NONE', *, *, #8998, .F. ) ;
#36095=EDGE_CURVE ( 'NONE', #30092, #43921, #10093, .T. ) ;
#36105=CARTESIAN_POINT ( 'NONE',  ( 0.1574803149606300023, -0.2714884749021748700, -1.284167712019357976 ) ) ;
#36107=VECTOR ( 'NONE', #47388, 39.37007874015748854 ) ;
#36128=CARTESIAN_POINT ( 'NONE',  ( -0.1476377952755905387, 0.4754249043493458116, -0.4843814799190158116 ) ) ;
#36175=ORIENTED_EDGE ( 'NONE', *, *, #22498, .F. ) ;
#36226=DIRECTION ( 'NONE',  ( -5.902779916321932142E-16, 0.2126700594527800581, -0.9771240687918557599 ) ) ;
#36233=ORIENTED_EDGE ( 'NONE', *, *, #29221, .T. ) ;
#36281=DIRECTION ( 'NONE',  ( 0.000000000000000000, -0.7880107536067207930, 0.6156614753256598460 ) ) ;
#36293=ORIENTED_EDGE ( 'NONE', *, *, #47402, .F. ) ;
#36386=CARTESIAN_POINT ( 'NONE',  ( -0.1574803149606299191, -0.9875035750853327077, -1.463737590216208861 ) ) ;
#36393=ADVANCED_FACE ( 'NONE', ( #21134 ), #42920, .T. ) ;
#36421=CARTESIAN_POINT ( 'NONE',  ( 0.1574803149606300023, 1.117014023967195735, -3.442880580079816788 ) ) ;
#36446=DIRECTION ( 'NONE',  ( 0.000000000000000000, -0.6156614753256628436, -0.7880107536067184615 ) ) ;
#36563=ORIENTED_EDGE ( 'NONE', *, *, #18701, .T. ) ;
#36585=DIRECTION ( 'NONE',  ( 0.000000000000000000, 0.7880107536067200158, -0.6156614753256608452 ) ) ;
#36612=LINE ( 'NONE', #3771, #32619 ) ;
#36622=ORIENTED_EDGE ( 'NONE', *, *, #4855, .F. ) ;
#36624=AXIS2_PLACEMENT_3D ( 'NONE', #26619, #8138, #41174 ) ;
#36657=DIRECTION ( 'NONE',  ( 0.000000000000000000, 0.000000000000000000, 1.000000000000000000 ) ) ;
#36681=TOROIDAL_SURFACE ( 'NONE', #26744, 0.3912448816427699927, 0.04921259842519685318 ) ;
#36789=AXIS2_PLACEMENT_3D ( 'NONE', #8594, #26836, #22984 ) ;
#36845=CARTESIAN_POINT ( 'NONE',  ( -0.1476377952755905387, 1.126631386849005878, -3.440787370833236380 ) ) ;
#36852=MECHANICAL_DESIGN_GEOMETRIC_PRESENTATION_REPRESENTATION('',(#33047),#23855);
#36871=AXIS2_PLACEMENT_3D ( 'NONE', #18545, #33201, #323 ) ;
#36874=CIRCLE ( 'NONE', #16238, 0.03937007874015748671 ) ;
#36883=AXIS2_PLACEMENT_3D ( 'NONE', #22069, #21355, #18478 ) ;
#36944=CARTESIAN_POINT ( 'NONE',  ( -0.1574803149606299191, 0.7443365962042343131, -3.523993443072799270 ) ) ;
#36982=DIRECTION ( 'NONE',  ( 0.000000000000000000, 0.000000000000000000, -1.000000000000000000 ) ) ;
#36983=ORIENTED_EDGE ( 'NONE', *, *, #24241, .T. ) ;
#36986=CARTESIAN_POINT ( 'NONE',  ( 0.1476377952755906220, -0.2237541348899639571, -1.272196386806235813 ) ) ;
#37013=DIRECTION ( 'NONE',  ( 0.000000000000000000, 0.6156614753256598460, 0.7880107536067207930 ) ) ;
#37045=EDGE_CURVE ( 'NONE', #46402, #25630, #16101, .T. ) ;
#37074=DIRECTION ( 'NONE',  ( 0.000000000000000000, 0.2126700594527834443, -0.9771240687918547607 ) ) ;
#37091=CYLINDRICAL_SURFACE ( 'NONE', #37102, 0.009842519685039378616 ) ;
#37102=AXIS2_PLACEMENT_3D ( 'NONE', #39966, #44039, #32589 ) ;
#37103=AXIS2_PLACEMENT_3D ( 'NONE', #6729, #25447, #21840 ) ;
#37146=ORIENTED_EDGE ( 'NONE', *, *, #13280, .F. ) ;
#37149=CARTESIAN_POINT ( 'NONE',  ( 0.1721082586868755704, -0.4313654725386900091, -0.9749915214042050859 ) ) ;
#37161=EDGE_CURVE ( 'NONE', #8495, #7550, #33960, .T. ) ;
#37244=CARTESIAN_POINT ( 'NONE',  ( -0.1594773935179923108, -0.4410959923581745379, -0.9673892061308028145 ) ) ;
#37272=LINE ( 'NONE', #22906, #22419 ) ;
#37300=CARTESIAN_POINT ( 'NONE',  ( 0.2066929133858268486, 0.5419727308409658662, -0.7545416139885202655 ) ) ;
#37377=CARTESIAN_POINT ( 'NONE',  ( 0.1992435948116500766, -0.3638053972758239496, -1.027775237132794173 ) ) ;
#37386=AXIS2_PLACEMENT_3D ( 'NONE', #46188, #28015, #42577 ) ;
#37402=CARTESIAN_POINT ( 'NONE',  ( -0.1574803149606299191, 0.07021257666615010606, -0.1553045758542774823 ) ) ;
#37450=FACE_OUTER_BOUND ( 'NONE', #18809, .T. ) ;
#37532=CARTESIAN_POINT ( 'NONE',  ( -0.2066929133858267931, -0.2237541348899638183, -1.272196386806236701 ) ) ;
#37557=AXIS2_PLACEMENT_3D ( 'NONE', #9790, #9074, #9557 ) ;
#37584=DIRECTION ( 'NONE',  ( 0.000000000000000000, -0.2432573283306646017, 0.9699617890481189164 ) ) ;
#37596=AXIS2_PLACEMENT_3D ( 'NONE', #28316, #21101, #32145 ) ;
#37624=CARTESIAN_POINT ( 'NONE',  ( 0.1574803149606300023, 1.126631386849005878, -3.440787370833236380 ) ) ;
#37633=ORIENTED_EDGE ( 'NONE', *, *, #39622, .T. ) ;
#37664=ORIENTED_EDGE ( 'NONE', *, *, #3086, .T. ) ;
#37712=LINE ( 'NONE', #33911, #13887 ) ;
#37740=CARTESIAN_POINT ( 'NONE',  ( -0.1574803149606299191, 1.117014023967196401, -3.442880580079819008 ) ) ;
#37749=ORIENTED_EDGE ( 'NONE', *, *, #13004, .T. ) ;
#37778=CARTESIAN_POINT ( 'NONE',  ( 0.1476377952755906220, -0.4075443641102559078, -0.9311509272141712534 ) ) ;
#37797=DIRECTION ( 'NONE',  ( 1.000000000000000000, 0.000000000000000000, 0.000000000000000000 ) ) ;
#37819=AXIS2_PLACEMENT_3D ( 'NONE', #42850, #35246, #2840 ) ;
#37824=CARTESIAN_POINT ( 'NONE',  ( 0.1476377952755906220, 1.126631386849005878, -3.440787370833236380 ) ) ;
#37846=DIRECTION ( 'NONE',  ( 1.000000000000000000, 0.000000000000000000, 0.000000000000000000 ) ) ;
#37929=CARTESIAN_POINT ( 'NONE',  ( 0.1574803149606300023, 0.09445121742700231249, -0.1242805304366906283 ) ) ;
#37947=EDGE_CURVE ( 'NONE', #41019, #24192, #11909, .T. ) ;
#37980=ORIENTED_EDGE ( 'NONE', *, *, #29447, .F. ) ;
#37986=EDGE_CURVE ( 'NONE', #5435, #34485, #15104, .T. ) ;
#38016=ORIENTED_EDGE ( 'NONE', *, *, #4855, .T. ) ;
#38039=CARTESIAN_POINT ( 'NONE',  ( 0.1673228346456693549, 0.09275486626281861935, -0.1104648588920805335 ) ) ;
#38052=EDGE_CURVE ( 'NONE', #7550, #20344, #27087, .T. ) ;
#38054=CARTESIAN_POINT ( 'NONE',  ( -0.1476377952755905387, 0.2573565155132549465, -0.3015174453633734930 ) ) ;
#38061=CARTESIAN_POINT ( 'NONE',  ( -0.2066929133858267931, 0.6201712226723911092, -1.113828806122273418 ) ) ;
#38063=ORIENTED_EDGE ( 'NONE', *, *, #41849, .F. ) ;
#38107=EDGE_CURVE ( 'NONE', #11278, #6310, #31055, .T. ) ;
#38110=DIMENSIONAL_EXPONENTS ( 1.000000000000000000, 0.000000000000000000, 0.000000000000000000, 0.000000000000000000, 0.000000000000000000, 0.000000000000000000, 0.000000000000000000 ) ;
#38117=DIRECTION ( 'NONE',  ( 0.000000000000000000, 0.2432573283306646017, -0.9699617890481189164 ) ) ;
#38249=ORIENTED_EDGE ( 'NONE', *, *, #5256, .F. ) ;
#38260=EDGE_CURVE ( 'NONE', #18185, #35433, #36612, .T. ) ;
#38272=FACE_OUTER_BOUND ( 'NONE', #27976, .T. ) ;
#38299=DIRECTION ( 'NONE',  ( 0.000000000000000000, 0.9699617890481186944, 0.2432573283306645462 ) ) ;
#38301=FACE_OUTER_BOUND ( 'NONE', #33450, .T. ) ;
#38306=ORIENTED_EDGE ( 'NONE', *, *, #38260, .T. ) ;
#38350=EDGE_CURVE ( 'NONE', #34485, #7195, #26496, .T. ) ;
#38410=VECTOR ( 'NONE', #21377, 39.37007874015748143 ) ;
#38423=CIRCLE ( 'NONE', #17763, 0.3912448816427701037 ) ;
#38442=FACE_OUTER_BOUND ( 'NONE', #10110, .T. ) ;
#38498=LINE ( 'NONE', #24137, #35205 ) ;
#38520=EDGE_LOOP ( 'NONE', ( #36983, #21704, #7498, #41761, #41763, #17739, #12958, #25650 ) ) ;
#38527=EDGE_CURVE ( 'NONE', #28221, #6831, #31076, .T. ) ;
#38636=EDGE_CURVE ( 'NONE', #18185, #8992, #33508, .T. ) ;
#38753=ORIENTED_EDGE ( 'NONE', *, *, #23116, .F. ) ;
#38784=CARTESIAN_POINT ( 'NONE',  ( 0.2066929133858268486, -0.9875035750853327077, -1.463737590216208861 ) ) ;
#38786=CARTESIAN_POINT ( 'NONE',  ( -0.2066929133858267931, -0.3022687907404924545, -1.075852903322848331 ) ) ;
#38794=ORIENTED_EDGE ( 'NONE', *, *, #39622, .F. ) ;
#38813=EDGE_CURVE ( 'NONE', #42574, #10554, #42521, .T. ) ;
#38979=CARTESIAN_POINT ( 'NONE',  ( 0.1476377952755906220, 0.06851622550196635741, -0.1414889043096673460 ) ) ;
#38983=AXIS2_PLACEMENT_3D ( 'NONE', #23748, #35723, #23998 ) ;
#39012=DIRECTION ( 'NONE',  ( -1.000000000000000000, -0.000000000000000000, 0.000000000000000000 ) ) ;
#39080=AXIS2_PLACEMENT_3D ( 'NONE', #44698, #8533, #36657 ) ;
#39111=ORIENTED_EDGE ( 'NONE', *, *, #17917, .F. ) ;
#39147=EDGE_LOOP ( 'NONE', ( #32876, #38063, #751, #38753 ) ) ;
#39149=VERTEX_POINT ( 'NONE', #809 ) ;
#39268=CLOSED_SHELL ( 'NONE', ( #44765, #32484, #1244, #13177, #43099, #8303, #3741, #3733, #16821, #2589, #1120, #44007, #3627, #17113, #5574, #29653, #11303, #26549, #1440, #47122, #23353, #4651, #41472, #32716, #32050, #12033, #1382, #39968, #9258, #28498, #28069, #33681, #32824, #16358, #47124, #13227, #43480, #15554, #18081, #32218, #12032, #41456, #4629, #35635, #9177, #46419, #5143, #22660, #44124, #33906, #5690, #24625, #35252, #44295, #36393, #42314, #16143, #46679, #2890, #13582 ) ) ;
#39270=ORIENTED_EDGE ( 'NONE', *, *, #23008, .T. ) ;
#39365=PLANE ( 'NONE',  #7500 ) ;
#39399=CARTESIAN_POINT ( 'NONE',  ( 0.1574803149606300023, -0.4008464425712924273, -0.9238935802775078976 ) ) ;
#39428=EDGE_CURVE ( 'NONE', #20344, #5435, #33413, .T. ) ;
#39429=ORIENTED_EDGE ( 'NONE', *, *, #9641, .F. ) ;
#39462=DIRECTION ( 'NONE',  ( 0.000000000000000000, 0.000000000000000000, 1.000000000000000000 ) ) ;
#39485=DIRECTION ( 'NONE',  ( -1.000000000000000000, -0.000000000000000000, 0.000000000000000000 ) ) ;
#39505=ORIENTED_EDGE ( 'NONE', *, *, #21130, .F. ) ;
#39549=CARTESIAN_POINT ( 'NONE',  ( -0.1476377952755905387, 0.7443365962042343131, -3.523993443072799270 ) ) ;
#39552=ORIENTED_EDGE ( 'NONE', *, *, #16994, .T. ) ;
#39557=ORIENTED_EDGE ( 'NONE', *, *, #28163, .T. ) ;
#39591=DIRECTION ( 'NONE',  ( 0.000000000000000000, -0.6156614753256597350, -0.7880107536067207930 ) ) ;
#39608=ORIENTED_EDGE ( 'NONE', *, *, #38052, .F. ) ;
#39622=EDGE_CURVE ( 'NONE', #26907, #28221, #22670, .T. ) ;
#39645=ORIENTED_EDGE ( 'NONE', *, *, #12295, .F. ) ;
#39661=AXIS2_PLACEMENT_3D ( 'NONE', #10676, #47322, #556 ) ;
#39665=VERTEX_POINT ( 'NONE', #266 ) ;
#39672=CIRCLE ( 'NONE', #34370, 0.7874015748031496509 ) ;
#39700=DIRECTION ( 'NONE',  ( 0.000000000000000000, -0.6156614753256566264, -0.7880107536067233465 ) ) ;
#39731=EDGE_CURVE ( 'NONE', #33099, #21515, #43512, .T. ) ;
#39739=EDGE_CURVE ( 'NONE', #45599, #5246, #44576, .T. ) ;
#39743=ORIENTED_EDGE ( 'NONE', *, *, #13233, .F. ) ;
#39747=PLANE ( 'NONE',  #26401 ) ;
#39944=VECTOR ( 'NONE', #35783, 39.37007874015748143 ) ;
#39965=CARTESIAN_POINT ( 'NONE',  ( -0.1574803149606299191, 0.2573565155132531146, -0.3015174453633728269 ) ) ;
#39966=CARTESIAN_POINT ( 'NONE',  ( -0.2066929133858267931, -0.4933358210236690744, -0.8766136318131756422 ) ) ;
#39968=ADVANCED_FACE ( 'NONE', ( #12923 ), #16009, .T. ) ;
#39970=VERTEX_POINT ( 'NONE', #45705 ) ;
#40013=LINE ( 'NONE', #3125, #45873 ) ;
#40055=DIRECTION ( 'NONE',  ( 0.000000000000000000, -0.7880107536067184615, 0.6156614753256628436 ) ) ;
#40085=CIRCLE ( 'NONE', #37819, 0.009842519685039371677 ) ;
#40111=CARTESIAN_POINT ( 'NONE',  ( 0.1476377952755906220, -0.2142072668875215635, -1.269802121763611291 ) ) ;
#40129=EDGE_CURVE ( 'NONE', #39970, #17877, #16449, .T. ) ;
#40143=ORIENTED_EDGE ( 'NONE', *, *, #13186, .F. ) ;
#40262=ORIENTED_EDGE ( 'NONE', *, *, #11700, .T. ) ;
#40263=CYLINDRICAL_SURFACE ( 'NONE', #36883, 0.009842519685039376881 ) ;
#40306=UNCERTAINTY_MEASURE_WITH_UNIT (LENGTH_MEASURE( 1.000000000000000082E-05 ), #1681, 'distance_accuracy_value', 'NONE') ;
#40324=DIRECTION ( 'NONE',  ( 0.000000000000000000, -9.251858538542971828E-16, 1.000000000000000000 ) ) ;
#40328=EDGE_CURVE ( 'NONE', #8597, #15230, #18326, .T. ) ;
#40336=DIRECTION ( 'NONE',  ( 0.000000000000000000, 0.9771240687918556489, 0.2126700594527800303 ) ) ;
#40339=CARTESIAN_POINT ( 'NONE',  ( -0.1574803149606299746, -0.4025872315894255538, -0.9257806984251616411 ) ) ;
#40442=CIRCLE ( 'NONE', #42728, 0.009842519685039376881 ) ;
#40490=FACE_OUTER_BOUND ( 'NONE', #47334, .T. ) ;
#40491=ORIENTED_EDGE ( 'NONE', *, *, #18184, .F. ) ;
#40500=ORIENTED_EDGE ( 'NONE', *, *, #1727, .F. ) ;
#40522=CYLINDRICAL_SURFACE ( 'NONE', #42236, 0.009842519685039491373 ) ;
#40524=ORIENTED_EDGE ( 'NONE', *, *, #24475, .F. ) ;
#40595=ORIENTED_EDGE ( 'NONE', *, *, #25154, .T. ) ;
#40679=CIRCLE ( 'NONE', #875, 0.7381889763779526659 ) ;
#40716=DIRECTION ( 'NONE',  ( -1.000000000000000000, -0.000000000000000000, -0.000000000000000000 ) ) ;
#40724=AXIS2_PLACEMENT_3D ( 'NONE', #31954, #6044, #36005 ) ;
#40793=SHAPE_DEFINITION_REPRESENTATION ( #31612, #5950 ) ;
#40813=CARTESIAN_POINT ( 'NONE',  ( -0.2066929133858267931, 0.5257908685547681982, -0.4487896632427120225 ) ) ;
#40814=ORIENTED_EDGE ( 'NONE', *, *, #21297, .F. ) ;
#40830=FILL_AREA_STYLE ('',( #23767 ) ) ;
#40859=CARTESIAN_POINT ( 'NONE',  ( 0.1968503937007874682, 0.06245656531175292070, -0.1492449156640645314 ) ) ;
#40881=ORIENTED_EDGE ( 'NONE', *, *, #32097, .T. ) ;
#40942=CYLINDRICAL_SURFACE ( 'NONE', #26684, 0.009842519685039378616 ) ;
#40947=DIRECTION ( 'NONE',  ( 0.000000000000000000, 0.9771240687918556489, 0.2126700594527794475 ) ) ;
#40975=EDGE_CURVE ( 'NONE', #12211, #30513, #19460, .T. ) ;
#40987=CARTESIAN_POINT ( 'NONE',  ( 0.1574803149606300023, 0.07021257666614877380, -0.1553045758542775656 ) ) ;
#41019=VERTEX_POINT ( 'NONE', #6706 ) ;
#41047=DIRECTION ( 'NONE',  ( 0.000000000000000000, 0.000000000000000000, 1.000000000000000000 ) ) ;
#41065=( BOUNDED_CURVE ( )  B_SPLINE_CURVE ( 3, ( #5924, #20542, #35177, #2325 ),
 .UNSPECIFIED., .F., .T. ) 
 B_SPLINE_CURVE_WITH_KNOTS ( ( 4, 4 ),
 ( 4.712388980384691450, 6.283185307179586232 ),
 .UNSPECIFIED. ) 
 CURVE ( )  GEOMETRIC_REPRESENTATION_ITEM ( )  RATIONAL_B_SPLINE_CURVE ( ( 1.000000000000000000, 0.8047378541243654926, 0.8047378541243654926, 1.000000000000000000 ) ) 
 REPRESENTATION_ITEM ( '' )  ) ;
#41114=CARTESIAN_POINT ( 'NONE',  ( 0.1574803149606300023, -0.2274162997038010614, -0.9219983537151217323 ) ) ;
#41123=CARTESIAN_POINT ( 'NONE',  ( -0.1564152455350579229, -0.4043437102334737077, -0.9276840032373354639 ) ) ;
#41126=DIRECTION ( 'NONE',  ( 0.000000000000000000, -0.6156614753256598460, -0.7880107536067207930 ) ) ;
#41155=EDGE_LOOP ( 'NONE', ( #24772, #29533, #17380, #16532 ) ) ;
#41156=LINE ( 'NONE', #34261, #24540 ) ;
#41157=VERTEX_POINT ( 'NONE', #44225 ) ;
#41165=DIRECTION ( 'NONE',  ( 0.000000000000000000, -0.6156614753256597350, -0.7880107536067206819 ) ) ;
#41174=DIRECTION ( 'NONE',  ( 0.000000000000000000, 0.000000000000000000, 1.000000000000000000 ) ) ;
#41243=EDGE_LOOP ( 'NONE', ( #23893, #45856, #16572, #34629 ) ) ;
#41277=CARTESIAN_POINT ( 'NONE',  ( 0.1574803149606300023, 1.571700394971587755, -2.465016072061059660 ) ) ;
#41282=CARTESIAN_POINT ( 'NONE',  ( -0.2056127690347618886, -0.3270319903728449717, -1.056505771383774661 ) ) ;
#41333=FACE_OUTER_BOUND ( 'NONE', #46865, .T. ) ;
#41403=VECTOR ( 'NONE', #22197, 39.37007874015748854 ) ;
#41456=ADVANCED_FACE ( 'NONE', ( #28481 ), #17201, .F. ) ;
#41472=ADVANCED_FACE ( 'NONE', ( #14800 ), #25820, .T. ) ;
#41499=AXIS2_PLACEMENT_3D ( 'NONE', #44344, #18720, #23690 ) ;
#41517=FACE_OUTER_BOUND ( 'NONE', #16360, .T. ) ;
#41572=ORIENTED_EDGE ( 'NONE', *, *, #2783, .F. ) ;
#41648=ORIENTED_EDGE ( 'NONE', *, *, #38813, .T. ) ;
#41676=SHAPE_REPRESENTATION_RELATIONSHIP ( 'NONE' , 'NONE' ,  #5950, #32480 ) ;
#41691=CARTESIAN_POINT ( 'NONE',  ( 0.1574803149606300023, 0.2876548164643194516, -0.2627373885913887319 ) ) ;
#41708=DIRECTION ( 'NONE',  ( 0.000000000000000000, 0.9771240687918550938, 0.2126700594527823895 ) ) ;
#41712=CARTESIAN_POINT ( 'NONE',  ( -0.1574803149606299191, 1.174718201258053041, -3.430321324600322797 ) ) ;
#41724=DIRECTION ( 'NONE',  ( 1.000000000000000000, -0.000000000000000000, -0.000000000000000000 ) ) ;
#41761=ORIENTED_EDGE ( 'NONE', *, *, #18239, .T. ) ;
#41763=ORIENTED_EDGE ( 'NONE', *, *, #847, .T. ) ;
#41767=CARTESIAN_POINT ( 'NONE',  ( 0.1574803149606300023, 1.174718201258053041, -3.430321324600322797 ) ) ;
#41772=DIRECTION ( 'NONE',  ( 0.000000000000000000, 6.938893903907222856E-15, -1.000000000000000000 ) ) ;
#41811=DIRECTION ( 'NONE',  ( 1.000000000000000000, 0.000000000000000000, 0.000000000000000000 ) ) ;
#41835=ORIENTED_EDGE ( 'NONE', *, *, #40975, .T. ) ;
#41841=DIRECTION ( 'NONE',  ( 0.000000000000000000, 0.7880107536067203489, -0.6156614753256602901 ) ) ;
#41849=EDGE_CURVE ( 'NONE', #8597, #5132, #11895, .T. ) ;
#41995=AXIS2_PLACEMENT_3D ( 'NONE', #18397, #30173, #19090 ) ;
#42029=DIRECTION ( 'NONE',  ( 0.000000000000000000, 0.9771240687918556489, 0.2126700594527794475 ) ) ;
#42085=CARTESIAN_POINT ( 'NONE',  ( 0.1574803149606299746, -0.2714884749021747590, -1.284167712019358198 ) ) ;
#42093=AXIS2_PLACEMENT_3D ( 'NONE', #30184, #8318, #11704 ) ;
#42094=DIRECTION ( 'NONE',  ( 0.000000000000000000, 0.000000000000000000, -1.000000000000000000 ) ) ;
#42095=CARTESIAN_POINT ( 'NONE',  ( -0.1476377952755905387, -0.9875035750853327077, -1.463737590216208861 ) ) ;
#42120=EDGE_CURVE ( 'NONE', #19153, #6659, #25079, .T. ) ;
#42135=AXIS2_PLACEMENT_3D ( 'NONE', #1518, #27452, #24299 ) ;
#42177=DIRECTION ( 'NONE',  ( 0.000000000000000000, 0.2432573283306931344, -0.9699617890481117000 ) ) ;
#42200=ORIENTED_EDGE ( 'NONE', *, *, #38527, .T. ) ;
#42211=FACE_OUTER_BOUND ( 'NONE', #22873, .T. ) ;
#42235=AXIS2_PLACEMENT_3D ( 'NONE', #25750, #7743, #36982 ) ;
#42236=AXIS2_PLACEMENT_3D ( 'NONE', #7712, #40055, #15399 ) ;
#42270=VECTOR ( 'NONE', #33608, 39.37007874015748143 ) ;
#42314=ADVANCED_FACE ( 'NONE', ( #44739 ), #29512, .T. ) ;
#42331=ORIENTED_EDGE ( 'NONE', *, *, #42871, .F. ) ;
#42333=CARTESIAN_POINT ( 'NONE',  ( -0.2066929133858267931, 0.7443365962042343131, -3.523993443072799270 ) ) ;
#42387=AXIS2_PLACEMENT_3D ( 'NONE', #33541, #43575, #25398 ) ;
#42397=VERTEX_POINT ( 'NONE', #1607 ) ;
#42400=DIRECTION ( 'NONE',  ( -1.000000000000000000, -0.000000000000000000, 0.000000000000000000 ) ) ;
#42462=VECTOR ( 'NONE', #2371, 39.37007874015748854 ) ;
#42485=DIRECTION ( 'NONE',  ( 0.000000000000000000, 0.000000000000000000, 1.000000000000000000 ) ) ;
#42504=CIRCLE ( 'NONE', #25687, 0.009842519685039330044 ) ;
#42506=ORIENTED_EDGE ( 'NONE', *, *, #15612, .T. ) ;
#42521=CIRCLE ( 'NONE', #20350, 0.009842519685039428923 ) ;
#42540=ORIENTED_EDGE ( 'NONE', *, *, #42120, .T. ) ;
#42550=ORIENTED_EDGE ( 'NONE', *, *, #10572, .F. ) ;
#42561=EDGE_LOOP ( 'NONE', ( #46099, #29436, #26377, #36089 ) ) ;
#42574=VERTEX_POINT ( 'NONE', #19239 ) ;
#42575=CARTESIAN_POINT ( 'NONE',  ( -0.1476377952755905387, -0.2142072668875215635, -1.269802121763611291 ) ) ;
#42577=DIRECTION ( 'NONE',  ( 0.000000000000000000, 0.000000000000000000, 1.000000000000000000 ) ) ;
#42614=DIRECTION ( 'NONE',  ( 0.000000000000000000, 0.7880107536067203489, -0.6156614753256602901 ) ) ;
#42685=DIRECTION ( 'NONE',  ( -0.000000000000000000, -0.2126700594527834443, 0.9771240687918547607 ) ) ;
#42697=ORIENTED_EDGE ( 'NONE', *, *, #35660, .T. ) ;
#42726=CARTESIAN_POINT ( 'NONE',  ( -0.1476377952755905387, 0.5323553679591567223, -0.7566348232351032266 ) ) ;
#42728=AXIS2_PLACEMENT_3D ( 'NONE', #22918, #44934, #19320 ) ;
#42850=CARTESIAN_POINT ( 'NONE',  ( -0.1476377952755905387, 0.06415291647593697466, -0.1630605872086743346 ) ) ;
#42871=EDGE_CURVE ( 'NONE', #25724, #30092, #42504, .T. ) ;
#42898=CIRCLE ( 'NONE', #37557, 0.7381889763779526659 ) ;
#42905=AXIS2_PLACEMENT_3D ( 'NONE', #15573, #37584, #23222 ) ;
#42920=CYLINDRICAL_SURFACE ( 'NONE', #10900, 0.009842519685039378616 ) ;
#42965=ORIENTED_EDGE ( 'NONE', *, *, #30668, .F. ) ;
#43031=ORIENTED_EDGE ( 'NONE', *, *, #13397, .T. ) ;
#43039=CIRCLE ( 'NONE', #44574, 0.04921259842519688094 ) ;
#43044=CARTESIAN_POINT ( 'NONE',  ( -0.1476377952755905387, -0.5010918323780657602, -0.8705539716229625524 ) ) ;
#43057=LINE ( 'NONE', #3763, #36107 ) ;
#43091=CARTESIAN_POINT ( 'NONE',  ( 0.1673228346456693549, 0.1005108776172154716, -0.1165245190822937205 ) ) ;
#43099=ADVANCED_FACE ( 'NONE', ( #20071 ), #23918, .T. ) ;
#43105=ORIENTED_EDGE ( 'NONE', *, *, #14679, .T. ) ;
#43116=ORIENTED_EDGE ( 'NONE', *, *, #3254, .F. ) ;
#43181=LINE ( 'NONE', #36013, #39944 ) ;
#43203=CARTESIAN_POINT ( 'NONE',  ( -0.2066929133858267931, -0.5192708129487060287, -0.8938220056861537755 ) ) ;
#43252=AXIS2_PLACEMENT_3D ( 'NONE', #1885, #39012, #9799 ) ;
#43273=CARTESIAN_POINT ( 'NONE',  ( -0.1574803149606299191, -0.4410959923581754816, -0.9673892061308019263 ) ) ;
#43306=CARTESIAN_POINT ( 'NONE',  ( -0.2066929133858267931, -0.9875035750853327077, -1.463737590216208861 ) ) ;
#43327=EDGE_CURVE ( 'NONE', #16549, #35433, #41065, .T. ) ;
#43405=CARTESIAN_POINT ( 'NONE',  ( -0.2066929133858267931, 0.09445121742700231249, -0.1242805304366906144 ) ) ;
#43407=CARTESIAN_POINT ( 'NONE',  ( 0.1574803149606299746, -0.4872761608334559846, -0.8688576204587790119 ) ) ;
#43476=DIRECTION ( 'NONE',  ( -1.000000000000000000, -0.000000000000000000, 0.000000000000000000 ) ) ;
#43480=ADVANCED_FACE ( 'NONE', ( #32541 ), #34916, .F. ) ;
#43489=CARTESIAN_POINT ( 'NONE',  ( -0.1574803149606299191, 0.05639690512153988644, -0.1570009270184609673 ) ) ;
#43512=CIRCLE ( 'NONE', #23653, 0.03937007874015748671 ) ;
#43537=DIRECTION ( 'NONE',  ( -0.000000000000000000, 0.7880107536067184615, -0.6156614753256628436 ) ) ;
#43575=DIRECTION ( 'NONE',  ( 1.000000000000000000, 0.000000000000000000, -0.000000000000000000 ) ) ;
#43605=VERTEX_POINT ( 'NONE', #19948 ) ;
#43616=FACE_OUTER_BOUND ( 'NONE', #43970, .T. ) ;
#43620=CARTESIAN_POINT ( 'NONE',  ( -0.1476377952755905387, -0.4889725119976394141, -0.8550419489141689589 ) ) ;
#43701=AXIS2_PLACEMENT_3D ( 'NONE', #4992, #16275, #45463 ) ;
#43758=CARTESIAN_POINT ( 'NONE',  ( -0.2066929133858267931, 0.7443365962042343131, -3.523993443072799270 ) ) ;
#43783=ORIENTED_EDGE ( 'NONE', *, *, #26913, .F. ) ;
#43786=AXIS2_PLACEMENT_3D ( 'NONE', #2915, #14676, #11556 ) ;
#43787=LINE ( 'NONE', #44242, #32886 ) ;
#43921=VERTEX_POINT ( 'NONE', #10369 ) ;
#43968=DIRECTION ( 'NONE',  ( -0.000000000000000000, -0.7880107536067200158, 0.6156614753256608452 ) ) ;
#43970=EDGE_LOOP ( 'NONE', ( #41648, #36293, #34239, #28582 ) ) ;
#44007=ADVANCED_FACE ( 'NONE', ( #3153 ), #10611, .F. ) ;
#44032=LINE ( 'NONE', #11001, #18604 ) ;
#44038=DIRECTION ( 'NONE',  ( 0.000000000000000000, 0.000000000000000000, -1.000000000000000000 ) ) ;
#44039=DIRECTION ( 'NONE',  ( 1.000000000000000000, 0.000000000000000000, 0.000000000000000000 ) ) ;
#44120=DIRECTION ( 'NONE',  ( 0.000000000000000000, -0.7880107536067207930, 0.6156614753256597350 ) ) ;
#44124=ADVANCED_FACE ( 'NONE', ( #28277 ), #28054, .T. ) ;
#44152=ORIENTED_EDGE ( 'NONE', *, *, #14197, .F. ) ;
#44188=CARTESIAN_POINT ( 'NONE',  ( -0.1775997780303593676, -0.4232972401690973108, -0.9812951153858839870 ) ) ;
#44191=FACE_OUTER_BOUND ( 'NONE', #3203, .T. ) ;
#44225=CARTESIAN_POINT ( 'NONE',  ( 0.1476377952755906220, 0.07021257666615010606, -0.1553045758542774823 ) ) ;
#44230=DIRECTION ( 'NONE',  ( 0.000000000000000000, -0.6156614753256584027, -0.7880107536067220142 ) ) ;
#44242=CARTESIAN_POINT ( 'NONE',  ( -0.1574803149606299191, -0.4014847039200427070, -0.9233949158597744011 ) ) ;
#44295=ADVANCED_FACE ( 'NONE', ( #14828 ), #37091, .T. ) ;
#44318=AXIS2_PLACEMENT_3D ( 'NONE', #40987, #30495, #12266 ) ;
#44338=DIRECTION ( 'NONE',  ( 0.000000000000000000, 0.000000000000000000, 1.000000000000000000 ) ) ;
#44344=CARTESIAN_POINT ( 'NONE',  ( -0.2066929133858267931, -0.5253304731389190074, -0.9015780170405504057 ) ) ;
#44347=ORIENTED_EDGE ( 'NONE', *, *, #34007, .T. ) ;
#44378=DIRECTION ( 'NONE',  ( 0.000000000000000000, 0.000000000000000000, -1.000000000000000000 ) ) ;
#44438=CARTESIAN_POINT ( 'NONE',  ( 0.1574803149606299746, 0.7443365962042343131, -3.964450923140766303 ) ) ;
#44447=CARTESIAN_POINT ( 'NONE',  ( -0.1574803149606299191, -0.2714884749021747590, -1.284167712019358198 ) ) ;
#44454=CIRCLE ( 'NONE', #20012, 0.7874015748031496509 ) ;
#44477=CARTESIAN_POINT ( 'NONE',  ( 0.1574803149606300023, -0.2237541348899642346, -1.272196386806234925 ) ) ;
#44479=DIRECTION ( 'NONE',  ( 1.000000000000000000, 0.000000000000000000, 0.000000000000000000 ) ) ;
#44545=FACE_OUTER_BOUND ( 'NONE', #41243, .T. ) ;
#44549=VECTOR ( 'NONE', #33085, 39.37007874015748143 ) ;
#44567=EDGE_CURVE ( 'NONE', #9478, #29301, #25680, .T. ) ;
#44574=AXIS2_PLACEMENT_3D ( 'NONE', #19215, #19686, #41708 ) ;
#44576=LINE ( 'NONE', #15628, #30552 ) ;
#44605=ORIENTED_EDGE ( 'NONE', *, *, #264, .T. ) ;
#44611=VERTEX_POINT ( 'NONE', #16253 ) ;
#44639=CARTESIAN_POINT ( 'NONE',  ( -0.1574803149606299191, -0.4008464425712929824, -0.9238935802775073425 ) ) ;
#44643=CARTESIAN_POINT ( 'NONE',  ( 0.2066929133858268486, 0.3648440108500937140, -3.619166627704267114 ) ) ;
#44698=CARTESIAN_POINT ( 'NONE',  ( 0.1574803149606300023, -0.2274162997038010614, -0.9219983537151217323 ) ) ;
#44704=CARTESIAN_POINT ( 'NONE',  ( 0.2066929133858268486, 0.2573565155132531701, -0.3015174453633727714 ) ) ;
#44713=CIRCLE ( 'NONE', #37103, 0.04921259842519686012 ) ;
#44714=CYLINDRICAL_SURFACE ( 'NONE', #34410, 0.7874015748031497619 ) ;
#44739=FACE_OUTER_BOUND ( 'NONE', #15467, .T. ) ;
#44740=ORIENTED_EDGE ( 'NONE', *, *, #23614, .F. ) ;
#44761=CARTESIAN_POINT ( 'NONE',  ( -0.2066929133858267931, -0.9654866319674424435, -1.480939111413832610 ) ) ;
#44765=ADVANCED_FACE ( 'NONE', ( #2548 ), #6137, .T. ) ;
#44817=DIRECTION ( 'NONE',  ( 1.000000000000000000, 0.000000000000000000, -0.000000000000000000 ) ) ;
#44934=DIRECTION ( 'NONE',  ( -7.005971165215254420E-15, 0.7880107536067203489, -0.6156614753256602901 ) ) ;
#44964=DIRECTION ( 'NONE',  ( 0.000000000000000000, -0.6156614753256619554, -0.7880107536067190166 ) ) ;
#44997=ORIENTED_EDGE ( 'NONE', *, *, #4046, .F. ) ;
#45003=DIRECTION ( 'NONE',  ( -1.000000000000000000, -0.000000000000000000, -0.000000000000000000 ) ) ;
#45104=VECTOR ( 'NONE', #21831, 39.37007874015748854 ) ;
#45117=VERTEX_POINT ( 'NONE', #38979 ) ;
#45119=DIRECTION ( 'NONE',  ( 0.000000000000000000, 0.000000000000000000, 1.000000000000000000 ) ) ;
#45204=CARTESIAN_POINT ( 'NONE',  ( -0.1968503937007874127, 0.07021257666614941217, -0.1553045758542781762 ) ) ;
#45245=DIRECTION ( 'NONE',  ( 0.000000000000000000, 0.000000000000000000, 1.000000000000000000 ) ) ;
#45253=EDGE_LOOP ( 'NONE', ( #42506, #37980, #39645, #4598, #30254 ) ) ;
#45307=DIRECTION ( 'NONE',  ( 0.000000000000000000, 0.9699617890481115889, 0.2432573283306930789 ) ) ;
#45335=ORIENTED_EDGE ( 'NONE', *, *, #4967, .T. ) ;
#45340=AXIS2_PLACEMENT_3D ( 'NONE', #7023, #36281, #3432 ) ;
#45370=EDGE_LOOP ( 'NONE', ( #28782, #24656, #16691, #18051 ) ) ;
#45386=EDGE_CURVE ( 'NONE', #28305, #17869, #32296, .T. ) ;
#45433=CARTESIAN_POINT ( 'NONE',  ( -0.1574803149606299191, 0.2512968553230417457, -0.3092734567177703453 ) ) ;
#45438=EDGE_CURVE ( 'NONE', #6624, #5180, #7107, .T. ) ;
#45442=FACE_OUTER_BOUND ( 'NONE', #25608, .T. ) ;
#45463=DIRECTION ( 'NONE',  ( 0.000000000000000000, -0.6156614753256597350, -0.7880107536067206819 ) ) ;
#45490=ORIENTED_EDGE ( 'NONE', *, *, #39428, .F. ) ;
#45514=VECTOR ( 'NONE', #40716, 39.37007874015748143 ) ;
#45517=FACE_OUTER_BOUND ( 'NONE', #30948, .T. ) ;
#45562=AXIS2_PLACEMENT_3D ( 'NONE', #32077, #33036, #39700 ) ;
#45599=VERTEX_POINT ( 'NONE', #12377 ) ;
#45625=ORIENTED_EDGE ( 'NONE', *, *, #15382, .T. ) ;
#45649=FACE_OUTER_BOUND ( 'NONE', #20002, .T. ) ;
#45672=ORIENTED_EDGE ( 'NONE', *, *, #28416, .F. ) ;
#45675=CARTESIAN_POINT ( 'NONE',  ( 0.1476377952755906220, -0.2274162997038010614, -0.9219983537151217323 ) ) ;
#45705=CARTESIAN_POINT ( 'NONE',  ( -0.1574803149606299191, -0.2142072668875218688, -1.269802121763611291 ) ) ;
#45725=EDGE_LOOP ( 'NONE', ( #21589, #8915, #26355, #37146 ) ) ;
#45762=TOROIDAL_SURFACE ( 'NONE', #36624, 0.7874015748031495399, 0.04921259842519685318 ) ;
#45772=CARTESIAN_POINT ( 'NONE',  ( 0.1476377952755906220, 1.117014023967196179, -3.442880580079819008 ) ) ;
#45856=ORIENTED_EDGE ( 'NONE', *, *, #33481, .F. ) ;
#45868=ORIENTED_EDGE ( 'NONE', *, *, #29496, .T. ) ;
#45873=VECTOR ( 'NONE', #18230, 39.37007874015748143 ) ;
#45920=LINE ( 'NONE', #17400, #8316 ) ;
#45932=ORIENTED_EDGE ( 'NONE', *, *, #29221, .F. ) ;
#45946=ORIENTED_EDGE ( 'NONE', *, *, #28416, .T. ) ;
#45985=CIRCLE ( 'NONE', #46726, 0.04921259842519686706 ) ;
#45991=EDGE_CURVE ( 'NONE', #6659, #8964, #40679, .T. ) ;
#46070=CIRCLE ( 'NONE', #40724, 0.009842519685039378616 ) ;
#46099=ORIENTED_EDGE ( 'NONE', *, *, #31942, .F. ) ;
#46101=AXIS2_PLACEMENT_3D ( 'NONE', #12050, #1705, #30509 ) ;
#46114=PRODUCT ( 'Link Bar', 'Link Bar', '', ( #11606 ) ) ;
#46175=CARTESIAN_POINT ( 'NONE',  ( -0.1574803149606299191, -0.2274162997038010614, -0.9219983537151217323 ) ) ;
#46188=CARTESIAN_POINT ( 'NONE',  ( -0.1574803149606299191, -0.2274162997038020051, -0.9219983537151217323 ) ) ;
#46211=DIRECTION ( 'NONE',  ( 1.110632647060516814E-14, -0.2432573283306702361, 0.9699617890481173621 ) ) ;
#46238=DIRECTION ( 'NONE',  ( 0.000000000000000000, 0.000000000000000000, 1.000000000000000000 ) ) ;
#46309=CIRCLE ( 'NONE', #19537, 0.7775590551181102983 ) ;
#46323=ORIENTED_EDGE ( 'NONE', *, *, #11700, .F. ) ;
#46334=VERTEX_POINT ( 'NONE', #8451 ) ;
#46345=ORIENTED_EDGE ( 'NONE', *, *, #27805, .F. ) ;
#46360=LINE ( 'NONE', #10192, #12382 ) ;
#46402=VERTEX_POINT ( 'NONE', #9650 ) ;
#46419=ADVANCED_FACE ( 'NONE', ( #42211 ), #26194, .T. ) ;
#46437=UNCERTAINTY_MEASURE_WITH_UNIT (LENGTH_MEASURE( 1.000000000000000082E-05 ), #34333, 'distance_accuracy_value', 'NONE') ;
#46482=ORIENTED_EDGE ( 'NONE', *, *, #38636, .F. ) ;
#46483=CARTESIAN_POINT ( 'NONE',  ( -0.2066929133858267931, 0.07021257666614935666, -0.1553045758542782318 ) ) ;
#46517=DIRECTION ( 'NONE',  ( 0.000000000000000000, 0.000000000000000000, 1.000000000000000000 ) ) ;
#46583=VECTOR ( 'NONE', #18786, 39.37007874015748854 ) ;
#46596=CYLINDRICAL_SURFACE ( 'NONE', #22850, 0.04921259842519686706 ) ;
#46601=DIRECTION ( 'NONE',  ( 0.000000000000000000, 0.6156614753256632877, 0.7880107536067181284 ) ) ;
#46606=EDGE_LOOP ( 'NONE', ( #2665, #10565, #40814, #29351, #39111, #24670, #26034, #2238 ) ) ;
#46616=CIRCLE ( 'NONE', #1451, 0.009842519685039369942 ) ;
#46617=ORIENTED_EDGE ( 'NONE', *, *, #31942, .T. ) ;
#46679=ADVANCED_FACE ( 'NONE', ( #11075 ), #40263, .T. ) ;
#46722=CARTESIAN_POINT ( 'NONE',  ( 0.1574803149606300023, -0.4950321721878526704, -0.8627979602685659222 ) ) ;
#46726=AXIS2_PLACEMENT_3D ( 'NONE', #23230, #18664, #34032 ) ;
#46774=CARTESIAN_POINT ( 'NONE',  ( -0.1673228346456692994, -0.4889725119976395251, -0.8550419489141688478 ) ) ;
#46775=ORIENTED_EDGE ( 'NONE', *, *, #45991, .T. ) ;
#46784=CARTESIAN_POINT ( 'NONE',  ( 0.1476377952755906220, 0.05639690512153986562, -0.1570009270184611894 ) ) ;
#46856=ORIENTED_EDGE ( 'NONE', *, *, #35297, .F. ) ;
#46862=AXIS2_PLACEMENT_3D ( 'NONE', #3681, #766, #310 ) ;
#46865=EDGE_LOOP ( 'NONE', ( #20224, #42965, #6652, #33504 ) ) ;
#46882=TOROIDAL_SURFACE ( 'NONE', #45340, 0.01968503937007873988, 0.009842519685039369942 ) ;
#46901=DIRECTION ( 'NONE',  ( -1.000000000000000000, -0.000000000000000000, 0.000000000000000000 ) ) ;
#46916=ORIENTED_EDGE ( 'NONE', *, *, #27637, .F. ) ;
#46917=ORIENTED_EDGE ( 'NONE', *, *, #38636, .T. ) ;
#46918=DIRECTION ( 'NONE',  ( 0.000000000000000000, 0.000000000000000000, 1.000000000000000000 ) ) ;
#46961=EDGE_CURVE ( 'NONE', #1272, #39970, #23897, .T. ) ;
#46967=PLANE ( 'NONE',  #26776 ) ;
#47058=DIRECTION ( 'NONE',  ( 0.000000000000000000, 0.000000000000000000, 1.000000000000000000 ) ) ;
#47122=ADVANCED_FACE ( 'NONE', ( #37450 ), #22836, .T. ) ;
#47123=ORIENTED_EDGE ( 'NONE', *, *, #13186, .T. ) ;
#47124=ADVANCED_FACE ( 'NONE', ( #4140 ), #159, .F. ) ;
#47128=VERTEX_POINT ( 'NONE', #18304 ) ;
#47303=VERTEX_POINT ( 'NONE', #23321 ) ;
#47322=DIRECTION ( 'NONE',  ( 5.553163235302570029E-14, 0.2432573283306915246, -0.9699617890481121441 ) ) ;
#47334=EDGE_LOOP ( 'NONE', ( #43031, #42540, #40500, #18667 ) ) ;
#47388=DIRECTION ( 'NONE',  ( 0.000000000000000000, -0.2432573283306645462, 0.9699617890481188054 ) ) ;
#47401=AXIS2_PLACEMENT_3D ( 'NONE', #20388, #6004, #20624 ) ;
#47402=EDGE_CURVE ( 'NONE', #17877, #10554, #4742, .T. ) ;
#47455=DIRECTION ( 'NONE',  ( 0.000000000000000000, -0.2432573283306645462, 0.9699617890481188054 ) ) ;
ENDSEC;
END-ISO-10303-21;
